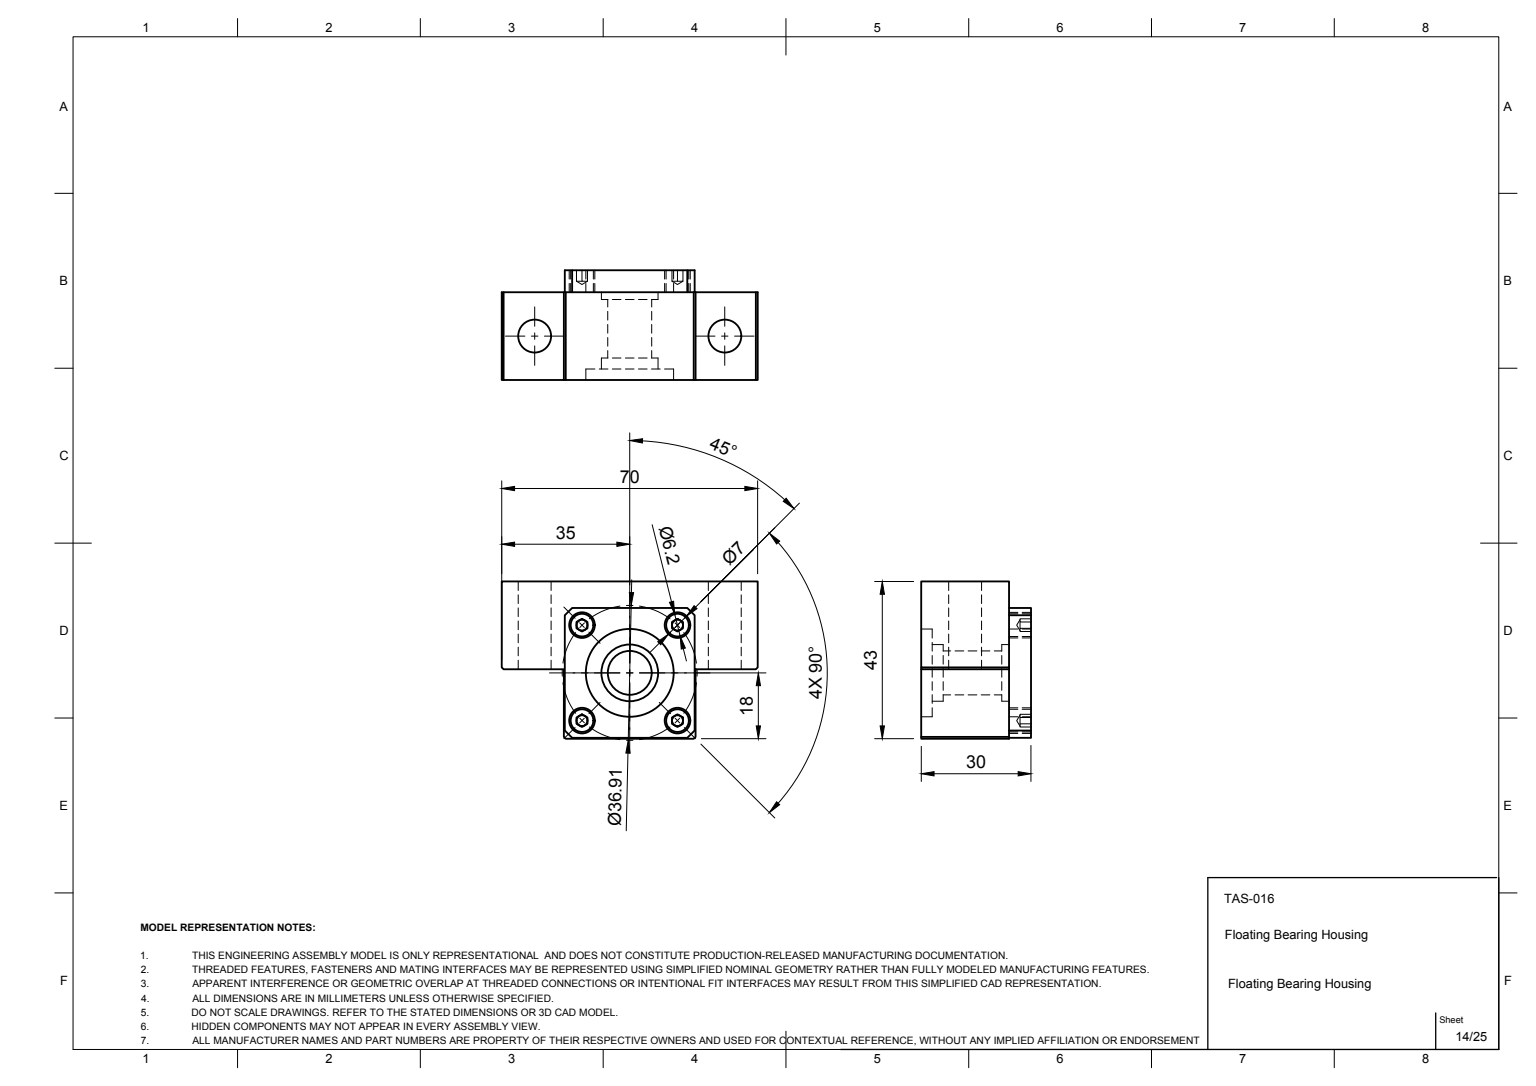
ISO-10303-21;
HEADER;
/* Generated by software containing ST-Developer
 * from STEP Tools, Inc. (www.steptools.com) 
 */

FILE_DESCRIPTION(
/* description */ ('STEP AP214'),
/* implementation_level */ '2;1');

FILE_NAME(
/* name */ 'Floating Bearing Housing.step',
/* time_stamp */ '2026-11-15T14:55:55-08:00',
/* author */ (''),
/* organization */ (''),
/* preprocessor_version */ 'ST-DEVELOPER v20.2',
/* originating_system */ 'Autodesk Translation Framework v15.17.0.0',
/* authorisation */ '');

FILE_SCHEMA (('AUTOMOTIVE_DESIGN { 1 0 10303 214 3 1 1 }'));
ENDSEC;

DATA;
#10=MECHANICAL_DESIGN_GEOMETRIC_PRESENTATION_REPRESENTATION('',(#929),#57079);
#871=SHAPE_REPRESENTATION_RELATIONSHIP('SRR','None',#57256,#900);
#900=ADVANCED_BREP_SHAPE_REPRESENTATION('',(#966),#57048);
#929=STYLED_ITEM('',(#57444),#966);
#966=MANIFOLD_SOLID_BREP('Body1',#24529);
#1046=FACE_BOUND('',#3680,.T.);
#1047=FACE_BOUND('',#3682,.T.);
#1048=FACE_BOUND('',#3684,.T.);
#1049=FACE_BOUND('',#3686,.T.);
#1050=FACE_BOUND('',#3688,.T.);
#1051=FACE_BOUND('',#3690,.T.);
#1052=FACE_BOUND('',#3694,.T.);
#1053=FACE_BOUND('',#3695,.T.);
#1054=FACE_BOUND('',#3699,.T.);
#1055=FACE_BOUND('',#3706,.T.);
#1056=FACE_BOUND('',#3708,.T.);
#1057=FACE_BOUND('',#3709,.T.);
#1058=FACE_BOUND('',#3710,.T.);
#1059=FACE_BOUND('',#3711,.T.);
#1060=FACE_BOUND('',#3712,.T.);
#1061=FACE_BOUND('',#3722,.T.);
#1062=FACE_BOUND('',#3724,.T.);
#1063=FACE_BOUND('',#3726,.T.);
#1064=FACE_BOUND('',#3728,.T.);
#1065=FACE_BOUND('',#3778,.T.);
#1066=FACE_BOUND('',#3780,.T.);
#1067=FACE_BOUND('',#3782,.T.);
#1068=FACE_BOUND('',#3784,.T.);
#1371=PLANE('',#25131);
#1372=PLANE('',#25132);
#1373=PLANE('',#25133);
#1374=PLANE('',#25134);
#1375=PLANE('',#25135);
#1376=PLANE('',#25136);
#1377=PLANE('',#25137);
#1378=PLANE('',#25138);
#1379=PLANE('',#25139);
#1380=PLANE('',#25140);
#1381=PLANE('',#25141);
#1382=PLANE('',#25142);
#1383=PLANE('',#25143);
#1384=PLANE('',#25144);
#1385=PLANE('',#25145);
#1386=PLANE('',#25146);
#1387=PLANE('',#25147);
#1388=PLANE('',#25148);
#1389=PLANE('',#25149);
#1390=PLANE('',#25150);
#1391=PLANE('',#25151);
#1392=PLANE('',#25152);
#1393=PLANE('',#25153);
#1394=PLANE('',#25154);
#1395=PLANE('',#25155);
#1396=PLANE('',#25156);
#1397=PLANE('',#25157);
#1398=PLANE('',#25158);
#1399=PLANE('',#25159);
#1400=PLANE('',#25160);
#1401=PLANE('',#25161);
#1402=PLANE('',#25162);
#1403=PLANE('',#25163);
#1404=PLANE('',#25164);
#1405=PLANE('',#25165);
#1406=PLANE('',#25166);
#1407=PLANE('',#25167);
#1408=PLANE('',#25168);
#1409=PLANE('',#25169);
#1410=PLANE('',#25170);
#1411=PLANE('',#25171);
#1412=PLANE('',#25172);
#1413=PLANE('',#25173);
#1414=PLANE('',#25174);
#1415=PLANE('',#25175);
#1416=PLANE('',#25176);
#1417=PLANE('',#25177);
#1418=PLANE('',#25178);
#1419=PLANE('',#25179);
#1420=PLANE('',#25180);
#1421=PLANE('',#25181);
#1422=PLANE('',#25182);
#1423=PLANE('',#25183);
#1424=PLANE('',#25184);
#1425=PLANE('',#25185);
#1426=PLANE('',#25186);
#1427=PLANE('',#25187);
#1428=PLANE('',#25188);
#1429=PLANE('',#25189);
#1430=PLANE('',#25190);
#1431=PLANE('',#25191);
#1432=PLANE('',#25192);
#1433=PLANE('',#25193);
#1434=PLANE('',#25194);
#1435=PLANE('',#25195);
#1436=PLANE('',#25196);
#1437=PLANE('',#25197);
#1438=PLANE('',#25198);
#1439=PLANE('',#25199);
#1440=PLANE('',#25200);
#1441=PLANE('',#25201);
#1442=PLANE('',#25202);
#1443=PLANE('',#25203);
#1444=PLANE('',#25204);
#1445=PLANE('',#25205);
#1446=PLANE('',#25206);
#1447=PLANE('',#25207);
#1448=PLANE('',#25208);
#1449=PLANE('',#25209);
#1450=PLANE('',#25210);
#1451=PLANE('',#25211);
#1452=PLANE('',#25212);
#1453=PLANE('',#25213);
#2114=CONICAL_SURFACE('',#25079,1.5,1.02974425867665);
#2115=CONICAL_SURFACE('',#25086,1.5,1.02974425867665);
#2116=CONICAL_SURFACE('',#25093,1.5,1.02974425867665);
#2117=CONICAL_SURFACE('',#25100,1.5,1.02974425867665);
#2239=FACE_OUTER_BOUND('',#3660,.T.);
#2240=FACE_OUTER_BOUND('',#3661,.T.);
#2241=FACE_OUTER_BOUND('',#3662,.T.);
#2242=FACE_OUTER_BOUND('',#3663,.T.);
#2243=FACE_OUTER_BOUND('',#3664,.T.);
#2244=FACE_OUTER_BOUND('',#3665,.T.);
#2245=FACE_OUTER_BOUND('',#3666,.T.);
#2246=FACE_OUTER_BOUND('',#3667,.T.);
#2247=FACE_OUTER_BOUND('',#3668,.T.);
#2248=FACE_OUTER_BOUND('',#3669,.T.);
#2249=FACE_OUTER_BOUND('',#3670,.T.);
#2250=FACE_OUTER_BOUND('',#3671,.T.);
#2251=FACE_OUTER_BOUND('',#3672,.T.);
#2252=FACE_OUTER_BOUND('',#3673,.T.);
#2253=FACE_OUTER_BOUND('',#3674,.T.);
#2254=FACE_OUTER_BOUND('',#3675,.T.);
#2255=FACE_OUTER_BOUND('',#3676,.T.);
#2256=FACE_OUTER_BOUND('',#3677,.T.);
#2257=FACE_OUTER_BOUND('',#3678,.T.);
#2258=FACE_OUTER_BOUND('',#3679,.T.);
#2259=FACE_OUTER_BOUND('',#3681,.T.);
#2260=FACE_OUTER_BOUND('',#3683,.T.);
#2261=FACE_OUTER_BOUND('',#3685,.T.);
#2262=FACE_OUTER_BOUND('',#3687,.T.);
#2263=FACE_OUTER_BOUND('',#3689,.T.);
#2264=FACE_OUTER_BOUND('',#3691,.T.);
#2265=FACE_OUTER_BOUND('',#3692,.T.);
#2266=FACE_OUTER_BOUND('',#3693,.T.);
#2267=FACE_OUTER_BOUND('',#3696,.T.);
#2268=FACE_OUTER_BOUND('',#3697,.T.);
#2269=FACE_OUTER_BOUND('',#3698,.T.);
#2270=FACE_OUTER_BOUND('',#3700,.T.);
#2271=FACE_OUTER_BOUND('',#3701,.T.);
#2272=FACE_OUTER_BOUND('',#3702,.T.);
#2273=FACE_OUTER_BOUND('',#3703,.T.);
#2274=FACE_OUTER_BOUND('',#3704,.T.);
#2275=FACE_OUTER_BOUND('',#3705,.T.);
#2276=FACE_OUTER_BOUND('',#3707,.T.);
#2277=FACE_OUTER_BOUND('',#3713,.T.);
#2278=FACE_OUTER_BOUND('',#3714,.T.);
#2279=FACE_OUTER_BOUND('',#3715,.T.);
#2280=FACE_OUTER_BOUND('',#3716,.T.);
#2281=FACE_OUTER_BOUND('',#3717,.T.);
#2282=FACE_OUTER_BOUND('',#3718,.T.);
#2283=FACE_OUTER_BOUND('',#3719,.T.);
#2284=FACE_OUTER_BOUND('',#3720,.T.);
#2285=FACE_OUTER_BOUND('',#3721,.T.);
#2286=FACE_OUTER_BOUND('',#3723,.T.);
#2287=FACE_OUTER_BOUND('',#3725,.T.);
#2288=FACE_OUTER_BOUND('',#3727,.T.);
#2289=FACE_OUTER_BOUND('',#3729,.T.);
#2290=FACE_OUTER_BOUND('',#3730,.T.);
#2291=FACE_OUTER_BOUND('',#3731,.T.);
#2292=FACE_OUTER_BOUND('',#3732,.T.);
#2293=FACE_OUTER_BOUND('',#3733,.T.);
#2294=FACE_OUTER_BOUND('',#3734,.T.);
#2295=FACE_OUTER_BOUND('',#3735,.T.);
#2296=FACE_OUTER_BOUND('',#3736,.T.);
#2297=FACE_OUTER_BOUND('',#3737,.T.);
#2298=FACE_OUTER_BOUND('',#3738,.T.);
#2299=FACE_OUTER_BOUND('',#3739,.T.);
#2300=FACE_OUTER_BOUND('',#3740,.T.);
#2301=FACE_OUTER_BOUND('',#3741,.T.);
#2302=FACE_OUTER_BOUND('',#3742,.T.);
#2303=FACE_OUTER_BOUND('',#3743,.T.);
#2304=FACE_OUTER_BOUND('',#3744,.T.);
#2305=FACE_OUTER_BOUND('',#3745,.T.);
#2306=FACE_OUTER_BOUND('',#3746,.T.);
#2307=FACE_OUTER_BOUND('',#3747,.T.);
#2308=FACE_OUTER_BOUND('',#3748,.T.);
#2309=FACE_OUTER_BOUND('',#3749,.T.);
#2310=FACE_OUTER_BOUND('',#3750,.T.);
#2311=FACE_OUTER_BOUND('',#3751,.T.);
#2312=FACE_OUTER_BOUND('',#3752,.T.);
#2313=FACE_OUTER_BOUND('',#3753,.T.);
#2314=FACE_OUTER_BOUND('',#3754,.T.);
#2315=FACE_OUTER_BOUND('',#3755,.T.);
#2316=FACE_OUTER_BOUND('',#3756,.T.);
#2317=FACE_OUTER_BOUND('',#3757,.T.);
#2318=FACE_OUTER_BOUND('',#3758,.T.);
#2319=FACE_OUTER_BOUND('',#3759,.T.);
#2320=FACE_OUTER_BOUND('',#3760,.T.);
#2321=FACE_OUTER_BOUND('',#3761,.T.);
#2322=FACE_OUTER_BOUND('',#3762,.T.);
#2323=FACE_OUTER_BOUND('',#3763,.T.);
#2324=FACE_OUTER_BOUND('',#3764,.T.);
#2325=FACE_OUTER_BOUND('',#3765,.T.);
#2326=FACE_OUTER_BOUND('',#3766,.T.);
#2327=FACE_OUTER_BOUND('',#3767,.T.);
#2328=FACE_OUTER_BOUND('',#3768,.T.);
#2329=FACE_OUTER_BOUND('',#3769,.T.);
#2330=FACE_OUTER_BOUND('',#3770,.T.);
#2331=FACE_OUTER_BOUND('',#3771,.T.);
#2332=FACE_OUTER_BOUND('',#3772,.T.);
#2333=FACE_OUTER_BOUND('',#3773,.T.);
#2334=FACE_OUTER_BOUND('',#3774,.T.);
#2335=FACE_OUTER_BOUND('',#3775,.T.);
#2336=FACE_OUTER_BOUND('',#3776,.T.);
#2337=FACE_OUTER_BOUND('',#3777,.T.);
#2338=FACE_OUTER_BOUND('',#3779,.T.);
#2339=FACE_OUTER_BOUND('',#3781,.T.);
#2340=FACE_OUTER_BOUND('',#3783,.T.);
#3660=EDGE_LOOP('',(#16272,#16273,#16274,#16275));
#3661=EDGE_LOOP('',(#16276,#16277,#16278,#16279));
#3662=EDGE_LOOP('',(#16280,#16281,#16282,#16283));
#3663=EDGE_LOOP('',(#16284,#16285,#16286,#16287));
#3664=EDGE_LOOP('',(#16288,#16289,#16290,#16291));
#3665=EDGE_LOOP('',(#16292,#16293,#16294,#16295));
#3666=EDGE_LOOP('',(#16296,#16297,#16298,#16299));
#3667=EDGE_LOOP('',(#16300,#16301,#16302,#16303,#16304,#16305,#16306,#16307));
#3668=EDGE_LOOP('',(#16308,#16309,#16310,#16311,#16312,#16313,#16314,#16315));
#3669=EDGE_LOOP('',(#16316,#16317,#16318,#16319,#16320,#16321,#16322,#16323));
#3670=EDGE_LOOP('',(#16324,#16325,#16326,#16327,#16328,#16329,#16330,#16331));
#3671=EDGE_LOOP('',(#16332,#16333,#16334,#16335));
#3672=EDGE_LOOP('',(#16336,#16337,#16338,#16339));
#3673=EDGE_LOOP('',(#16340,#16341,#16342,#16343));
#3674=EDGE_LOOP('',(#16344,#16345,#16346,#16347));
#3675=EDGE_LOOP('',(#16348,#16349,#16350,#16351));
#3676=EDGE_LOOP('',(#16352,#16353,#16354,#16355));
#3677=EDGE_LOOP('',(#16356,#16357,#16358,#16359));
#3678=EDGE_LOOP('',(#16360,#16361,#16362,#16363));
#3679=EDGE_LOOP('',(#16364));
#3680=EDGE_LOOP('',(#16365));
#3681=EDGE_LOOP('',(#16366));
#3682=EDGE_LOOP('',(#16367));
#3683=EDGE_LOOP('',(#16368));
#3684=EDGE_LOOP('',(#16369));
#3685=EDGE_LOOP('',(#16370));
#3686=EDGE_LOOP('',(#16371));
#3687=EDGE_LOOP('',(#16372,#16373,#16374,#16375,#16376,#16377,#16378,#16379,
#16380,#16381,#16382,#16383));
#3688=EDGE_LOOP('',(#16384,#16385,#16386,#16387,#16388,#16389,#16390,#16391));
#3689=EDGE_LOOP('',(#16392,#16393,#16394,#16395));
#3690=EDGE_LOOP('',(#16396));
#3691=EDGE_LOOP('',(#16397,#16398,#16399,#16400));
#3692=EDGE_LOOP('',(#16401,#16402,#16403,#16404));
#3693=EDGE_LOOP('',(#16405,#16406,#16407,#16408));
#3694=EDGE_LOOP('',(#16409));
#3695=EDGE_LOOP('',(#16410));
#3696=EDGE_LOOP('',(#16411,#16412,#16413,#16414));
#3697=EDGE_LOOP('',(#16415,#16416,#16417,#16418));
#3698=EDGE_LOOP('',(#16419,#16420,#16421,#16422));
#3699=EDGE_LOOP('',(#16423));
#3700=EDGE_LOOP('',(#16424,#16425,#16426,#16427));
#3701=EDGE_LOOP('',(#16428,#16429,#16430,#16431));
#3702=EDGE_LOOP('',(#16432,#16433,#16434,#16435));
#3703=EDGE_LOOP('',(#16436,#16437,#16438,#16439));
#3704=EDGE_LOOP('',(#16440,#16441,#16442,#16443));
#3705=EDGE_LOOP('',(#16444,#16445,#16446,#16447,#16448,#16449,#16450,#16451,
#16452,#16453,#16454,#16455));
#3706=EDGE_LOOP('',(#16456));
#3707=EDGE_LOOP('',(#16457,#16458,#16459,#16460,#16461,#16462,#16463,#16464));
#3708=EDGE_LOOP('',(#16465));
#3709=EDGE_LOOP('',(#16466));
#3710=EDGE_LOOP('',(#16467));
#3711=EDGE_LOOP('',(#16468));
#3712=EDGE_LOOP('',(#16469));
#3713=EDGE_LOOP('',(#16470,#16471,#16472,#16473));
#3714=EDGE_LOOP('',(#16474,#16475,#16476,#16477));
#3715=EDGE_LOOP('',(#16478,#16479,#16480,#16481));
#3716=EDGE_LOOP('',(#16482,#16483,#16484,#16485));
#3717=EDGE_LOOP('',(#16486,#16487,#16488,#16489));
#3718=EDGE_LOOP('',(#16490,#16491,#16492,#16493));
#3719=EDGE_LOOP('',(#16494,#16495,#16496,#16497));
#3720=EDGE_LOOP('',(#16498,#16499,#16500,#16501));
#3721=EDGE_LOOP('',(#16502));
#3722=EDGE_LOOP('',(#16503,#16504,#16505,#16506,#16507,#16508));
#3723=EDGE_LOOP('',(#16509));
#3724=EDGE_LOOP('',(#16510,#16511,#16512,#16513,#16514,#16515));
#3725=EDGE_LOOP('',(#16516));
#3726=EDGE_LOOP('',(#16517,#16518,#16519,#16520,#16521,#16522));
#3727=EDGE_LOOP('',(#16523));
#3728=EDGE_LOOP('',(#16524,#16525,#16526,#16527,#16528,#16529));
#3729=EDGE_LOOP('',(#16530,#16531,#16532,#16533,#16534));
#3730=EDGE_LOOP('',(#16535,#16536,#16537,#16538,#16539));
#3731=EDGE_LOOP('',(#16540,#16541,#16542,#16543,#16544));
#3732=EDGE_LOOP('',(#16545,#16546,#16547,#16548,#16549));
#3733=EDGE_LOOP('',(#16550,#16551,#16552,#16553,#16554));
#3734=EDGE_LOOP('',(#16555,#16556,#16557,#16558,#16559));
#3735=EDGE_LOOP('',(#16560,#16561,#16562));
#3736=EDGE_LOOP('',(#16563,#16564,#16565));
#3737=EDGE_LOOP('',(#16566,#16567,#16568));
#3738=EDGE_LOOP('',(#16569,#16570,#16571));
#3739=EDGE_LOOP('',(#16572,#16573,#16574));
#3740=EDGE_LOOP('',(#16575,#16576,#16577));
#3741=EDGE_LOOP('',(#16578,#16579,#16580,#16581,#16582));
#3742=EDGE_LOOP('',(#16583,#16584,#16585,#16586,#16587));
#3743=EDGE_LOOP('',(#16588,#16589,#16590,#16591,#16592));
#3744=EDGE_LOOP('',(#16593,#16594,#16595,#16596,#16597));
#3745=EDGE_LOOP('',(#16598,#16599,#16600,#16601,#16602));
#3746=EDGE_LOOP('',(#16603,#16604,#16605,#16606,#16607));
#3747=EDGE_LOOP('',(#16608,#16609,#16610));
#3748=EDGE_LOOP('',(#16611,#16612,#16613));
#3749=EDGE_LOOP('',(#16614,#16615,#16616));
#3750=EDGE_LOOP('',(#16617,#16618,#16619));
#3751=EDGE_LOOP('',(#16620,#16621,#16622));
#3752=EDGE_LOOP('',(#16623,#16624,#16625));
#3753=EDGE_LOOP('',(#16626,#16627,#16628,#16629,#16630));
#3754=EDGE_LOOP('',(#16631,#16632,#16633,#16634,#16635));
#3755=EDGE_LOOP('',(#16636,#16637,#16638,#16639,#16640));
#3756=EDGE_LOOP('',(#16641,#16642,#16643,#16644,#16645));
#3757=EDGE_LOOP('',(#16646,#16647,#16648,#16649,#16650));
#3758=EDGE_LOOP('',(#16651,#16652,#16653,#16654,#16655));
#3759=EDGE_LOOP('',(#16656,#16657,#16658));
#3760=EDGE_LOOP('',(#16659,#16660,#16661));
#3761=EDGE_LOOP('',(#16662,#16663,#16664));
#3762=EDGE_LOOP('',(#16665,#16666,#16667));
#3763=EDGE_LOOP('',(#16668,#16669,#16670));
#3764=EDGE_LOOP('',(#16671,#16672,#16673));
#3765=EDGE_LOOP('',(#16674,#16675,#16676,#16677,#16678));
#3766=EDGE_LOOP('',(#16679,#16680,#16681,#16682,#16683));
#3767=EDGE_LOOP('',(#16684,#16685,#16686,#16687,#16688));
#3768=EDGE_LOOP('',(#16689,#16690,#16691,#16692,#16693));
#3769=EDGE_LOOP('',(#16694,#16695,#16696,#16697,#16698));
#3770=EDGE_LOOP('',(#16699,#16700,#16701,#16702,#16703));
#3771=EDGE_LOOP('',(#16704,#16705,#16706));
#3772=EDGE_LOOP('',(#16707,#16708,#16709));
#3773=EDGE_LOOP('',(#16710,#16711,#16712));
#3774=EDGE_LOOP('',(#16713,#16714,#16715));
#3775=EDGE_LOOP('',(#16716,#16717,#16718));
#3776=EDGE_LOOP('',(#16719,#16720,#16721));
#3777=EDGE_LOOP('',(#16722));
#3778=EDGE_LOOP('',(#16723));
#3779=EDGE_LOOP('',(#16724));
#3780=EDGE_LOOP('',(#16725));
#3781=EDGE_LOOP('',(#16726));
#3782=EDGE_LOOP('',(#16727));
#3783=EDGE_LOOP('',(#16728));
#3784=EDGE_LOOP('',(#16729));
#5331=LINE('',#35183,#7298);
#5332=LINE('',#35189,#7299);
#5333=LINE('',#35195,#7300);
#5334=LINE('',#35201,#7301);
#5335=LINE('',#35207,#7302);
#5336=LINE('',#35213,#7303);
#5337=LINE('',#35219,#7304);
#5338=LINE('',#35224,#7305);
#5339=LINE('',#35239,#7306);
#5340=LINE('',#35254,#7307);
#5341=LINE('',#35269,#7308);
#5342=LINE('',#35285,#7309);
#5343=LINE('',#35291,#7310);
#5344=LINE('',#35297,#7311);
#5345=LINE('',#35303,#7312);
#5346=LINE('',#35309,#7313);
#5347=LINE('',#35315,#7314);
#5348=LINE('',#35321,#7315);
#5349=LINE('',#35327,#7316);
#5350=LINE('',#35336,#7317);
#5351=LINE('',#35338,#7318);
#5352=LINE('',#35340,#7319);
#5353=LINE('',#35342,#7320);
#5354=LINE('',#35344,#7321);
#5355=LINE('',#35346,#7322);
#5356=LINE('',#35348,#7323);
#5357=LINE('',#35350,#7324);
#5358=LINE('',#35352,#7325);
#5359=LINE('',#35354,#7326);
#5360=LINE('',#35356,#7327);
#5361=LINE('',#35357,#7328);
#5362=LINE('',#35360,#7329);
#5363=LINE('',#35362,#7330);
#5364=LINE('',#35364,#7331);
#5365=LINE('',#35366,#7332);
#5366=LINE('',#35368,#7333);
#5367=LINE('',#35370,#7334);
#5368=LINE('',#35372,#7335);
#5369=LINE('',#35373,#7336);
#5370=LINE('',#35377,#7337);
#5371=LINE('',#35378,#7338);
#5372=LINE('',#35379,#7339);
#5373=LINE('',#35382,#7340);
#5374=LINE('',#35383,#7341);
#5375=LINE('',#35386,#7342);
#5376=LINE('',#35387,#7343);
#5377=LINE('',#35390,#7344);
#5378=LINE('',#35391,#7345);
#5379=LINE('',#35394,#7346);
#5380=LINE('',#35395,#7347);
#5381=LINE('',#35398,#7348);
#5382=LINE('',#35399,#7349);
#5383=LINE('',#35402,#7350);
#5384=LINE('',#35403,#7351);
#5385=LINE('',#35406,#7352);
#5386=LINE('',#35407,#7353);
#5387=LINE('',#35410,#7354);
#5388=LINE('',#35411,#7355);
#5389=LINE('',#35414,#7356);
#5390=LINE('',#35415,#7357);
#5391=LINE('',#35418,#7358);
#5392=LINE('',#35419,#7359);
#5393=LINE('',#35421,#7360);
#5394=LINE('',#35426,#7361);
#5395=LINE('',#35428,#7362);
#5396=LINE('',#35430,#7363);
#5397=LINE('',#35432,#7364);
#5398=LINE('',#35434,#7365);
#5399=LINE('',#35436,#7366);
#5400=LINE('',#35438,#7367);
#5401=LINE('',#35439,#7368);
#5402=LINE('',#35441,#7369);
#5403=LINE('',#35442,#7370);
#5404=LINE('',#35444,#7371);
#5405=LINE('',#35446,#7372);
#5406=LINE('',#35448,#7373);
#5407=LINE('',#35450,#7374);
#5408=LINE('',#35452,#7375);
#5409=LINE('',#35454,#7376);
#5410=LINE('',#35459,#7377);
#5411=LINE('',#35461,#7378);
#5412=LINE('',#35463,#7379);
#5413=LINE('',#35465,#7380);
#5414=LINE('',#35467,#7381);
#5415=LINE('',#35468,#7382);
#5416=LINE('',#35472,#7383);
#5417=LINE('',#35474,#7384);
#5418=LINE('',#35476,#7385);
#5419=LINE('',#35478,#7386);
#5420=LINE('',#35480,#7387);
#5421=LINE('',#35481,#7388);
#5422=LINE('',#35485,#7389);
#5423=LINE('',#35487,#7390);
#5424=LINE('',#35489,#7391);
#5425=LINE('',#35491,#7392);
#5426=LINE('',#35493,#7393);
#5427=LINE('',#35494,#7394);
#5428=LINE('',#35498,#7395);
#5429=LINE('',#35500,#7396);
#5430=LINE('',#35502,#7397);
#5431=LINE('',#35504,#7398);
#5432=LINE('',#35506,#7399);
#5433=LINE('',#35507,#7400);
#5434=LINE('',#35510,#7401);
#5435=LINE('',#35511,#7402);
#5436=LINE('',#35513,#7403);
#5437=LINE('',#35514,#7404);
#5438=LINE('',#35516,#7405);
#5439=LINE('',#35518,#7406);
#5440=LINE('',#35519,#7407);
#5441=LINE('',#35521,#7408);
#5442=LINE('',#35523,#7409);
#5443=LINE('',#35524,#7410);
#5444=LINE('',#35526,#7411);
#5445=LINE('',#35528,#7412);
#5446=LINE('',#35529,#7413);
#5447=LINE('',#35531,#7414);
#5448=LINE('',#35533,#7415);
#5449=LINE('',#35534,#7416);
#5450=LINE('',#35536,#7417);
#5451=LINE('',#35537,#7418);
#5452=LINE('',#35546,#7419);
#5453=LINE('',#35547,#7420);
#5454=LINE('',#35549,#7421);
#5455=LINE('',#35550,#7422);
#5456=LINE('',#35552,#7423);
#5457=LINE('',#35554,#7424);
#5458=LINE('',#35555,#7425);
#5459=LINE('',#35557,#7426);
#5460=LINE('',#35559,#7427);
#5461=LINE('',#35560,#7428);
#5462=LINE('',#35562,#7429);
#5463=LINE('',#35564,#7430);
#5464=LINE('',#35565,#7431);
#5465=LINE('',#35567,#7432);
#5466=LINE('',#35569,#7433);
#5467=LINE('',#35570,#7434);
#5468=LINE('',#35572,#7435);
#5469=LINE('',#35573,#7436);
#5470=LINE('',#35582,#7437);
#5471=LINE('',#35583,#7438);
#5472=LINE('',#35585,#7439);
#5473=LINE('',#35586,#7440);
#5474=LINE('',#35588,#7441);
#5475=LINE('',#35590,#7442);
#5476=LINE('',#35591,#7443);
#5477=LINE('',#35593,#7444);
#5478=LINE('',#35595,#7445);
#5479=LINE('',#35596,#7446);
#5480=LINE('',#35598,#7447);
#5481=LINE('',#35600,#7448);
#5482=LINE('',#35601,#7449);
#5483=LINE('',#35603,#7450);
#5484=LINE('',#35605,#7451);
#5485=LINE('',#35606,#7452);
#5486=LINE('',#35608,#7453);
#5487=LINE('',#35609,#7454);
#5488=LINE('',#35618,#7455);
#5489=LINE('',#35619,#7456);
#5490=LINE('',#35621,#7457);
#5491=LINE('',#35622,#7458);
#5492=LINE('',#35624,#7459);
#5493=LINE('',#35626,#7460);
#5494=LINE('',#35627,#7461);
#5495=LINE('',#35629,#7462);
#5496=LINE('',#35631,#7463);
#5497=LINE('',#35632,#7464);
#5498=LINE('',#35634,#7465);
#5499=LINE('',#35636,#7466);
#5500=LINE('',#35637,#7467);
#5501=LINE('',#35639,#7468);
#5502=LINE('',#35641,#7469);
#5503=LINE('',#35642,#7470);
#5504=LINE('',#35644,#7471);
#5505=LINE('',#35645,#7472);
#7298=VECTOR('',#27911,4.49999999999999);
#7299=VECTOR('',#27918,4.49999999999999);
#7300=VECTOR('',#27925,12.);
#7301=VECTOR('',#27932,7.75);
#7302=VECTOR('',#27939,6.);
#7303=VECTOR('',#27946,7.74999999999999);
#7304=VECTOR('',#27953,12.);
#7305=VECTOR('',#27958,1.5);
#7306=VECTOR('',#27973,1.5);
#7307=VECTOR('',#27988,1.5);
#7308=VECTOR('',#28003,1.5);
#7309=VECTOR('',#28020,3.1);
#7310=VECTOR('',#28027,3.1);
#7311=VECTOR('',#28034,3.1);
#7312=VECTOR('',#28041,3.1);
#7313=VECTOR('',#28048,3.5);
#7314=VECTOR('',#28055,3.5);
#7315=VECTOR('',#28062,3.50000000000001);
#7316=VECTOR('',#28069,3.50000000000001);
#7317=VECTOR('',#28082,1000.);
#7318=VECTOR('',#28083,1000.);
#7319=VECTOR('',#28084,1000.);
#7320=VECTOR('',#28085,1000.);
#7321=VECTOR('',#28086,1000.);
#7322=VECTOR('',#28087,1000.);
#7323=VECTOR('',#28088,1000.);
#7324=VECTOR('',#28089,1000.);
#7325=VECTOR('',#28090,1000.);
#7326=VECTOR('',#28091,1000.);
#7327=VECTOR('',#28092,1000.);
#7328=VECTOR('',#28093,1000.);
#7329=VECTOR('',#28094,1000.);
#7330=VECTOR('',#28095,1000.);
#7331=VECTOR('',#28096,1000.);
#7332=VECTOR('',#28097,1000.);
#7333=VECTOR('',#28098,1000.);
#7334=VECTOR('',#28099,1000.);
#7335=VECTOR('',#28100,1000.);
#7336=VECTOR('',#28101,1000.);
#7337=VECTOR('',#28104,1000.);
#7338=VECTOR('',#28105,1000.);
#7339=VECTOR('',#28106,1000.);
#7340=VECTOR('',#28109,1000.);
#7341=VECTOR('',#28110,1000.);
#7342=VECTOR('',#28113,1000.);
#7343=VECTOR('',#28114,1000.);
#7344=VECTOR('',#28117,1000.);
#7345=VECTOR('',#28118,1000.);
#7346=VECTOR('',#28121,1000.);
#7347=VECTOR('',#28122,1000.);
#7348=VECTOR('',#28125,1000.);
#7349=VECTOR('',#28126,1000.);
#7350=VECTOR('',#28129,1000.);
#7351=VECTOR('',#28130,1000.);
#7352=VECTOR('',#28133,1000.);
#7353=VECTOR('',#28134,1000.);
#7354=VECTOR('',#28137,1000.);
#7355=VECTOR('',#28138,1000.);
#7356=VECTOR('',#28141,1000.);
#7357=VECTOR('',#28142,1000.);
#7358=VECTOR('',#28145,1000.);
#7359=VECTOR('',#28146,1000.);
#7360=VECTOR('',#28149,1000.);
#7361=VECTOR('',#28154,1000.);
#7362=VECTOR('',#28155,1000.);
#7363=VECTOR('',#28156,1000.);
#7364=VECTOR('',#28157,1000.);
#7365=VECTOR('',#28158,1000.);
#7366=VECTOR('',#28159,1000.);
#7367=VECTOR('',#28160,1000.);
#7368=VECTOR('',#28161,1000.);
#7369=VECTOR('',#28164,1000.);
#7370=VECTOR('',#28165,1000.);
#7371=VECTOR('',#28168,1000.);
#7372=VECTOR('',#28171,1000.);
#7373=VECTOR('',#28174,1000.);
#7374=VECTOR('',#28177,1000.);
#7375=VECTOR('',#28180,1000.);
#7376=VECTOR('',#28183,1000.);
#7377=VECTOR('',#28188,1000.);
#7378=VECTOR('',#28189,1000.);
#7379=VECTOR('',#28190,1000.);
#7380=VECTOR('',#28191,1000.);
#7381=VECTOR('',#28192,1000.);
#7382=VECTOR('',#28193,1000.);
#7383=VECTOR('',#28196,1000.);
#7384=VECTOR('',#28197,1000.);
#7385=VECTOR('',#28198,1000.);
#7386=VECTOR('',#28199,1000.);
#7387=VECTOR('',#28200,1000.);
#7388=VECTOR('',#28201,1000.);
#7389=VECTOR('',#28204,1000.);
#7390=VECTOR('',#28205,1000.);
#7391=VECTOR('',#28206,1000.);
#7392=VECTOR('',#28207,1000.);
#7393=VECTOR('',#28208,1000.);
#7394=VECTOR('',#28209,1000.);
#7395=VECTOR('',#28212,1000.);
#7396=VECTOR('',#28213,1000.);
#7397=VECTOR('',#28214,1000.);
#7398=VECTOR('',#28215,1000.);
#7399=VECTOR('',#28216,1000.);
#7400=VECTOR('',#28217,1000.);
#7401=VECTOR('',#28220,1000.);
#7402=VECTOR('',#28221,1000.);
#7403=VECTOR('',#28222,1000.);
#7404=VECTOR('',#28223,1000.);
#7405=VECTOR('',#28226,1000.);
#7406=VECTOR('',#28227,1000.);
#7407=VECTOR('',#28228,1000.);
#7408=VECTOR('',#28231,1000.);
#7409=VECTOR('',#28232,1000.);
#7410=VECTOR('',#28233,1000.);
#7411=VECTOR('',#28236,1000.);
#7412=VECTOR('',#28237,1000.);
#7413=VECTOR('',#28238,1000.);
#7414=VECTOR('',#28241,1000.);
#7415=VECTOR('',#28242,1000.);
#7416=VECTOR('',#28243,1000.);
#7417=VECTOR('',#28246,1000.);
#7418=VECTOR('',#28247,1000.);
#7419=VECTOR('',#28262,1000.);
#7420=VECTOR('',#28263,1000.);
#7421=VECTOR('',#28264,1000.);
#7422=VECTOR('',#28265,1000.);
#7423=VECTOR('',#28268,1000.);
#7424=VECTOR('',#28269,1000.);
#7425=VECTOR('',#28270,1000.);
#7426=VECTOR('',#28273,1000.);
#7427=VECTOR('',#28274,1000.);
#7428=VECTOR('',#28275,1000.);
#7429=VECTOR('',#28278,1000.);
#7430=VECTOR('',#28279,1000.);
#7431=VECTOR('',#28280,1000.);
#7432=VECTOR('',#28283,1000.);
#7433=VECTOR('',#28284,1000.);
#7434=VECTOR('',#28285,1000.);
#7435=VECTOR('',#28288,1000.);
#7436=VECTOR('',#28289,1000.);
#7437=VECTOR('',#28304,1000.);
#7438=VECTOR('',#28305,1000.);
#7439=VECTOR('',#28306,1000.);
#7440=VECTOR('',#28307,1000.);
#7441=VECTOR('',#28310,1000.);
#7442=VECTOR('',#28311,1000.);
#7443=VECTOR('',#28312,1000.);
#7444=VECTOR('',#28315,1000.);
#7445=VECTOR('',#28316,1000.);
#7446=VECTOR('',#28317,1000.);
#7447=VECTOR('',#28320,1000.);
#7448=VECTOR('',#28321,1000.);
#7449=VECTOR('',#28322,1000.);
#7450=VECTOR('',#28325,1000.);
#7451=VECTOR('',#28326,1000.);
#7452=VECTOR('',#28327,1000.);
#7453=VECTOR('',#28330,1000.);
#7454=VECTOR('',#28331,1000.);
#7455=VECTOR('',#28346,1000.);
#7456=VECTOR('',#28347,1000.);
#7457=VECTOR('',#28348,1000.);
#7458=VECTOR('',#28349,1000.);
#7459=VECTOR('',#28352,1000.);
#7460=VECTOR('',#28353,1000.);
#7461=VECTOR('',#28354,1000.);
#7462=VECTOR('',#28357,1000.);
#7463=VECTOR('',#28358,1000.);
#7464=VECTOR('',#28359,1000.);
#7465=VECTOR('',#28362,1000.);
#7466=VECTOR('',#28363,1000.);
#7467=VECTOR('',#28364,1000.);
#7468=VECTOR('',#28367,1000.);
#7469=VECTOR('',#28368,1000.);
#7470=VECTOR('',#28369,1000.);
#7471=VECTOR('',#28372,1000.);
#7472=VECTOR('',#28373,1000.);
#9270=CIRCLE('',#25059,4.5);
#9271=CIRCLE('',#25060,4.49999999999999);
#9272=CIRCLE('',#25062,4.5);
#9273=CIRCLE('',#25063,4.49999999999999);
#9274=CIRCLE('',#25065,12.);
#9275=CIRCLE('',#25066,12.);
#9276=CIRCLE('',#25068,7.75);
#9277=CIRCLE('',#25069,7.74999999999999);
#9278=CIRCLE('',#25071,6.00000000000001);
#9279=CIRCLE('',#25072,6.00000000000001);
#9280=CIRCLE('',#25074,7.74999999999999);
#9281=CIRCLE('',#25075,7.74999999999999);
#9282=CIRCLE('',#25077,12.);
#9283=CIRCLE('',#25078,12.);
#9284=CIRCLE('',#25080,1.5);
#9285=CIRCLE('',#25081,1.5);
#9286=CIRCLE('',#25082,1.5);
#9287=CIRCLE('',#25083,1.5);
#9288=CIRCLE('',#25084,1.5);
#9289=CIRCLE('',#25085,1.5);
#9290=CIRCLE('',#25087,1.5);
#9291=CIRCLE('',#25088,1.5);
#9292=CIRCLE('',#25089,1.5);
#9293=CIRCLE('',#25090,1.5);
#9294=CIRCLE('',#25091,1.5);
#9295=CIRCLE('',#25092,1.5);
#9296=CIRCLE('',#25094,1.5);
#9297=CIRCLE('',#25095,1.5);
#9298=CIRCLE('',#25096,1.5);
#9299=CIRCLE('',#25097,1.5);
#9300=CIRCLE('',#25098,1.5);
#9301=CIRCLE('',#25099,1.5);
#9302=CIRCLE('',#25101,1.5);
#9303=CIRCLE('',#25102,1.5);
#9304=CIRCLE('',#25103,1.5);
#9305=CIRCLE('',#25104,1.5);
#9306=CIRCLE('',#25105,1.5);
#9307=CIRCLE('',#25106,1.5);
#9308=CIRCLE('',#25108,3.1);
#9309=CIRCLE('',#25109,3.1);
#9310=CIRCLE('',#25111,3.1);
#9311=CIRCLE('',#25112,3.1);
#9312=CIRCLE('',#25114,3.1);
#9313=CIRCLE('',#25115,3.1);
#9314=CIRCLE('',#25117,3.1);
#9315=CIRCLE('',#25118,3.1);
#9316=CIRCLE('',#25120,3.5);
#9317=CIRCLE('',#25121,3.5);
#9318=CIRCLE('',#25123,3.5);
#9319=CIRCLE('',#25124,3.5);
#9320=CIRCLE('',#25126,3.50000000000001);
#9321=CIRCLE('',#25127,3.50000000000001);
#9322=CIRCLE('',#25129,3.50000000000001);
#9323=CIRCLE('',#25130,3.50000000000001);
#10397=VERTEX_POINT('',#35180);
#10398=VERTEX_POINT('',#35182);
#10399=VERTEX_POINT('',#35186);
#10400=VERTEX_POINT('',#35188);
#10401=VERTEX_POINT('',#35192);
#10402=VERTEX_POINT('',#35194);
#10403=VERTEX_POINT('',#35198);
#10404=VERTEX_POINT('',#35200);
#10405=VERTEX_POINT('',#35204);
#10406=VERTEX_POINT('',#35206);
#10407=VERTEX_POINT('',#35210);
#10408=VERTEX_POINT('',#35212);
#10409=VERTEX_POINT('',#35216);
#10410=VERTEX_POINT('',#35218);
#10411=VERTEX_POINT('',#35222);
#10412=VERTEX_POINT('',#35223);
#10413=VERTEX_POINT('',#35225);
#10414=VERTEX_POINT('',#35227);
#10415=VERTEX_POINT('',#35229);
#10416=VERTEX_POINT('',#35231);
#10417=VERTEX_POINT('',#35233);
#10418=VERTEX_POINT('',#35237);
#10419=VERTEX_POINT('',#35238);
#10420=VERTEX_POINT('',#35240);
#10421=VERTEX_POINT('',#35242);
#10422=VERTEX_POINT('',#35244);
#10423=VERTEX_POINT('',#35246);
#10424=VERTEX_POINT('',#35248);
#10425=VERTEX_POINT('',#35252);
#10426=VERTEX_POINT('',#35253);
#10427=VERTEX_POINT('',#35255);
#10428=VERTEX_POINT('',#35257);
#10429=VERTEX_POINT('',#35259);
#10430=VERTEX_POINT('',#35261);
#10431=VERTEX_POINT('',#35263);
#10432=VERTEX_POINT('',#35267);
#10433=VERTEX_POINT('',#35268);
#10434=VERTEX_POINT('',#35270);
#10435=VERTEX_POINT('',#35272);
#10436=VERTEX_POINT('',#35274);
#10437=VERTEX_POINT('',#35276);
#10438=VERTEX_POINT('',#35278);
#10439=VERTEX_POINT('',#35282);
#10440=VERTEX_POINT('',#35284);
#10441=VERTEX_POINT('',#35288);
#10442=VERTEX_POINT('',#35290);
#10443=VERTEX_POINT('',#35294);
#10444=VERTEX_POINT('',#35296);
#10445=VERTEX_POINT('',#35300);
#10446=VERTEX_POINT('',#35302);
#10447=VERTEX_POINT('',#35306);
#10448=VERTEX_POINT('',#35308);
#10449=VERTEX_POINT('',#35312);
#10450=VERTEX_POINT('',#35314);
#10451=VERTEX_POINT('',#35318);
#10452=VERTEX_POINT('',#35320);
#10453=VERTEX_POINT('',#35324);
#10454=VERTEX_POINT('',#35326);
#10455=VERTEX_POINT('',#35334);
#10456=VERTEX_POINT('',#35335);
#10457=VERTEX_POINT('',#35337);
#10458=VERTEX_POINT('',#35339);
#10459=VERTEX_POINT('',#35341);
#10460=VERTEX_POINT('',#35343);
#10461=VERTEX_POINT('',#35345);
#10462=VERTEX_POINT('',#35347);
#10463=VERTEX_POINT('',#35349);
#10464=VERTEX_POINT('',#35351);
#10465=VERTEX_POINT('',#35353);
#10466=VERTEX_POINT('',#35355);
#10467=VERTEX_POINT('',#35358);
#10468=VERTEX_POINT('',#35359);
#10469=VERTEX_POINT('',#35361);
#10470=VERTEX_POINT('',#35363);
#10471=VERTEX_POINT('',#35365);
#10472=VERTEX_POINT('',#35367);
#10473=VERTEX_POINT('',#35369);
#10474=VERTEX_POINT('',#35371);
#10475=VERTEX_POINT('',#35375);
#10476=VERTEX_POINT('',#35376);
#10477=VERTEX_POINT('',#35381);
#10478=VERTEX_POINT('',#35385);
#10479=VERTEX_POINT('',#35389);
#10480=VERTEX_POINT('',#35393);
#10481=VERTEX_POINT('',#35397);
#10482=VERTEX_POINT('',#35401);
#10483=VERTEX_POINT('',#35405);
#10484=VERTEX_POINT('',#35409);
#10485=VERTEX_POINT('',#35413);
#10486=VERTEX_POINT('',#35417);
#10487=VERTEX_POINT('',#35424);
#10488=VERTEX_POINT('',#35425);
#10489=VERTEX_POINT('',#35427);
#10490=VERTEX_POINT('',#35429);
#10491=VERTEX_POINT('',#35431);
#10492=VERTEX_POINT('',#35433);
#10493=VERTEX_POINT('',#35435);
#10494=VERTEX_POINT('',#35437);
#10495=VERTEX_POINT('',#35457);
#10496=VERTEX_POINT('',#35458);
#10497=VERTEX_POINT('',#35460);
#10498=VERTEX_POINT('',#35462);
#10499=VERTEX_POINT('',#35464);
#10500=VERTEX_POINT('',#35466);
#10501=VERTEX_POINT('',#35470);
#10502=VERTEX_POINT('',#35471);
#10503=VERTEX_POINT('',#35473);
#10504=VERTEX_POINT('',#35475);
#10505=VERTEX_POINT('',#35477);
#10506=VERTEX_POINT('',#35479);
#10507=VERTEX_POINT('',#35483);
#10508=VERTEX_POINT('',#35484);
#10509=VERTEX_POINT('',#35486);
#10510=VERTEX_POINT('',#35488);
#10511=VERTEX_POINT('',#35490);
#10512=VERTEX_POINT('',#35492);
#10513=VERTEX_POINT('',#35496);
#10514=VERTEX_POINT('',#35497);
#10515=VERTEX_POINT('',#35499);
#10516=VERTEX_POINT('',#35501);
#10517=VERTEX_POINT('',#35503);
#10518=VERTEX_POINT('',#35505);
#10519=VERTEX_POINT('',#35509);
#10520=VERTEX_POINT('',#35512);
#10521=VERTEX_POINT('',#35517);
#10522=VERTEX_POINT('',#35522);
#10523=VERTEX_POINT('',#35527);
#10524=VERTEX_POINT('',#35532);
#10525=VERTEX_POINT('',#35545);
#10526=VERTEX_POINT('',#35548);
#10527=VERTEX_POINT('',#35553);
#10528=VERTEX_POINT('',#35558);
#10529=VERTEX_POINT('',#35563);
#10530=VERTEX_POINT('',#35568);
#10531=VERTEX_POINT('',#35581);
#10532=VERTEX_POINT('',#35584);
#10533=VERTEX_POINT('',#35589);
#10534=VERTEX_POINT('',#35594);
#10535=VERTEX_POINT('',#35599);
#10536=VERTEX_POINT('',#35604);
#10537=VERTEX_POINT('',#35617);
#10538=VERTEX_POINT('',#35620);
#10539=VERTEX_POINT('',#35625);
#10540=VERTEX_POINT('',#35630);
#10541=VERTEX_POINT('',#35635);
#10542=VERTEX_POINT('',#35640);
#12681=EDGE_CURVE('',#10397,#10397,#9270,.T.);
#12682=EDGE_CURVE('',#10397,#10398,#5331,.T.);
#12683=EDGE_CURVE('',#10398,#10398,#9271,.T.);
#12684=EDGE_CURVE('',#10399,#10399,#9272,.T.);
#12685=EDGE_CURVE('',#10399,#10400,#5332,.T.);
#12686=EDGE_CURVE('',#10400,#10400,#9273,.T.);
#12687=EDGE_CURVE('',#10401,#10401,#9274,.T.);
#12688=EDGE_CURVE('',#10401,#10402,#5333,.T.);
#12689=EDGE_CURVE('',#10402,#10402,#9275,.T.);
#12690=EDGE_CURVE('',#10403,#10403,#9276,.T.);
#12691=EDGE_CURVE('',#10403,#10404,#5334,.T.);
#12692=EDGE_CURVE('',#10404,#10404,#9277,.T.);
#12693=EDGE_CURVE('',#10405,#10405,#9278,.T.);
#12694=EDGE_CURVE('',#10405,#10406,#5335,.T.);
#12695=EDGE_CURVE('',#10406,#10406,#9279,.T.);
#12696=EDGE_CURVE('',#10407,#10407,#9280,.T.);
#12697=EDGE_CURVE('',#10407,#10408,#5336,.T.);
#12698=EDGE_CURVE('',#10408,#10408,#9281,.T.);
#12699=EDGE_CURVE('',#10409,#10409,#9282,.T.);
#12700=EDGE_CURVE('',#10409,#10410,#5337,.T.);
#12701=EDGE_CURVE('',#10410,#10410,#9283,.T.);
#12702=EDGE_CURVE('',#10411,#10412,#5338,.T.);
#12703=EDGE_CURVE('',#10412,#10413,#9284,.T.);
#12704=EDGE_CURVE('',#10413,#10414,#9285,.T.);
#12705=EDGE_CURVE('',#10414,#10415,#9286,.T.);
#12706=EDGE_CURVE('',#10415,#10416,#9287,.T.);
#12707=EDGE_CURVE('',#10416,#10417,#9288,.T.);
#12708=EDGE_CURVE('',#10417,#10412,#9289,.T.);
#12709=EDGE_CURVE('',#10418,#10419,#5339,.T.);
#12710=EDGE_CURVE('',#10419,#10420,#9290,.T.);
#12711=EDGE_CURVE('',#10420,#10421,#9291,.T.);
#12712=EDGE_CURVE('',#10421,#10422,#9292,.T.);
#12713=EDGE_CURVE('',#10422,#10423,#9293,.T.);
#12714=EDGE_CURVE('',#10423,#10424,#9294,.T.);
#12715=EDGE_CURVE('',#10424,#10419,#9295,.T.);
#12716=EDGE_CURVE('',#10425,#10426,#5340,.T.);
#12717=EDGE_CURVE('',#10426,#10427,#9296,.T.);
#12718=EDGE_CURVE('',#10427,#10428,#9297,.T.);
#12719=EDGE_CURVE('',#10428,#10429,#9298,.T.);
#12720=EDGE_CURVE('',#10429,#10430,#9299,.T.);
#12721=EDGE_CURVE('',#10430,#10431,#9300,.T.);
#12722=EDGE_CURVE('',#10431,#10426,#9301,.T.);
#12723=EDGE_CURVE('',#10432,#10433,#5341,.T.);
#12724=EDGE_CURVE('',#10433,#10434,#9302,.T.);
#12725=EDGE_CURVE('',#10434,#10435,#9303,.T.);
#12726=EDGE_CURVE('',#10435,#10436,#9304,.T.);
#12727=EDGE_CURVE('',#10436,#10437,#9305,.T.);
#12728=EDGE_CURVE('',#10437,#10438,#9306,.T.);
#12729=EDGE_CURVE('',#10438,#10433,#9307,.T.);
#12730=EDGE_CURVE('',#10439,#10439,#9308,.T.);
#12731=EDGE_CURVE('',#10439,#10440,#5342,.T.);
#12732=EDGE_CURVE('',#10440,#10440,#9309,.T.);
#12733=EDGE_CURVE('',#10441,#10441,#9310,.T.);
#12734=EDGE_CURVE('',#10441,#10442,#5343,.T.);
#12735=EDGE_CURVE('',#10442,#10442,#9311,.T.);
#12736=EDGE_CURVE('',#10443,#10443,#9312,.T.);
#12737=EDGE_CURVE('',#10443,#10444,#5344,.T.);
#12738=EDGE_CURVE('',#10444,#10444,#9313,.T.);
#12739=EDGE_CURVE('',#10445,#10445,#9314,.T.);
#12740=EDGE_CURVE('',#10445,#10446,#5345,.T.);
#12741=EDGE_CURVE('',#10446,#10446,#9315,.T.);
#12742=EDGE_CURVE('',#10447,#10447,#9316,.T.);
#12743=EDGE_CURVE('',#10447,#10448,#5346,.T.);
#12744=EDGE_CURVE('',#10448,#10448,#9317,.T.);
#12745=EDGE_CURVE('',#10449,#10449,#9318,.T.);
#12746=EDGE_CURVE('',#10449,#10450,#5347,.T.);
#12747=EDGE_CURVE('',#10450,#10450,#9319,.T.);
#12748=EDGE_CURVE('',#10451,#10451,#9320,.T.);
#12749=EDGE_CURVE('',#10451,#10452,#5348,.T.);
#12750=EDGE_CURVE('',#10452,#10452,#9321,.T.);
#12751=EDGE_CURVE('',#10453,#10453,#9322,.T.);
#12752=EDGE_CURVE('',#10453,#10454,#5349,.T.);
#12753=EDGE_CURVE('',#10454,#10454,#9323,.T.);
#12754=EDGE_CURVE('',#10455,#10456,#5350,.T.);
#12755=EDGE_CURVE('',#10456,#10457,#5351,.T.);
#12756=EDGE_CURVE('',#10457,#10458,#5352,.T.);
#12757=EDGE_CURVE('',#10458,#10459,#5353,.T.);
#12758=EDGE_CURVE('',#10459,#10460,#5354,.T.);
#12759=EDGE_CURVE('',#10460,#10461,#5355,.T.);
#12760=EDGE_CURVE('',#10461,#10462,#5356,.T.);
#12761=EDGE_CURVE('',#10462,#10463,#5357,.T.);
#12762=EDGE_CURVE('',#10463,#10464,#5358,.T.);
#12763=EDGE_CURVE('',#10464,#10465,#5359,.T.);
#12764=EDGE_CURVE('',#10465,#10466,#5360,.T.);
#12765=EDGE_CURVE('',#10466,#10455,#5361,.T.);
#12766=EDGE_CURVE('',#10467,#10468,#5362,.T.);
#12767=EDGE_CURVE('',#10469,#10467,#5363,.T.);
#12768=EDGE_CURVE('',#10470,#10469,#5364,.T.);
#12769=EDGE_CURVE('',#10471,#10470,#5365,.T.);
#12770=EDGE_CURVE('',#10472,#10471,#5366,.T.);
#12771=EDGE_CURVE('',#10473,#10472,#5367,.T.);
#12772=EDGE_CURVE('',#10474,#10473,#5368,.T.);
#12773=EDGE_CURVE('',#10468,#10474,#5369,.T.);
#12774=EDGE_CURVE('',#10475,#10476,#5370,.T.);
#12775=EDGE_CURVE('',#10456,#10476,#5371,.T.);
#12776=EDGE_CURVE('',#10455,#10475,#5372,.T.);
#12777=EDGE_CURVE('',#10476,#10477,#5373,.T.);
#12778=EDGE_CURVE('',#10457,#10477,#5374,.T.);
#12779=EDGE_CURVE('',#10477,#10478,#5375,.T.);
#12780=EDGE_CURVE('',#10458,#10478,#5376,.T.);
#12781=EDGE_CURVE('',#10478,#10479,#5377,.T.);
#12782=EDGE_CURVE('',#10459,#10479,#5378,.T.);
#12783=EDGE_CURVE('',#10479,#10480,#5379,.T.);
#12784=EDGE_CURVE('',#10460,#10480,#5380,.T.);
#12785=EDGE_CURVE('',#10480,#10481,#5381,.T.);
#12786=EDGE_CURVE('',#10461,#10481,#5382,.T.);
#12787=EDGE_CURVE('',#10481,#10482,#5383,.T.);
#12788=EDGE_CURVE('',#10462,#10482,#5384,.T.);
#12789=EDGE_CURVE('',#10482,#10483,#5385,.T.);
#12790=EDGE_CURVE('',#10463,#10483,#5386,.T.);
#12791=EDGE_CURVE('',#10483,#10484,#5387,.T.);
#12792=EDGE_CURVE('',#10464,#10484,#5388,.T.);
#12793=EDGE_CURVE('',#10484,#10485,#5389,.T.);
#12794=EDGE_CURVE('',#10465,#10485,#5390,.T.);
#12795=EDGE_CURVE('',#10485,#10486,#5391,.T.);
#12796=EDGE_CURVE('',#10466,#10486,#5392,.T.);
#12797=EDGE_CURVE('',#10486,#10475,#5393,.T.);
#12798=EDGE_CURVE('',#10487,#10488,#5394,.T.);
#12799=EDGE_CURVE('',#10488,#10489,#5395,.T.);
#12800=EDGE_CURVE('',#10489,#10490,#5396,.T.);
#12801=EDGE_CURVE('',#10490,#10491,#5397,.T.);
#12802=EDGE_CURVE('',#10491,#10492,#5398,.T.);
#12803=EDGE_CURVE('',#10492,#10493,#5399,.T.);
#12804=EDGE_CURVE('',#10493,#10494,#5400,.T.);
#12805=EDGE_CURVE('',#10494,#10487,#5401,.T.);
#12806=EDGE_CURVE('',#10488,#10467,#5402,.T.);
#12807=EDGE_CURVE('',#10487,#10469,#5403,.T.);
#12808=EDGE_CURVE('',#10489,#10468,#5404,.T.);
#12809=EDGE_CURVE('',#10490,#10474,#5405,.T.);
#12810=EDGE_CURVE('',#10491,#10473,#5406,.T.);
#12811=EDGE_CURVE('',#10492,#10472,#5407,.T.);
#12812=EDGE_CURVE('',#10493,#10471,#5408,.T.);
#12813=EDGE_CURVE('',#10494,#10470,#5409,.T.);
#12814=EDGE_CURVE('',#10495,#10496,#5410,.T.);
#12815=EDGE_CURVE('',#10497,#10495,#5411,.T.);
#12816=EDGE_CURVE('',#10498,#10497,#5412,.T.);
#12817=EDGE_CURVE('',#10499,#10498,#5413,.T.);
#12818=EDGE_CURVE('',#10500,#10499,#5414,.T.);
#12819=EDGE_CURVE('',#10496,#10500,#5415,.T.);
#12820=EDGE_CURVE('',#10501,#10502,#5416,.T.);
#12821=EDGE_CURVE('',#10503,#10501,#5417,.T.);
#12822=EDGE_CURVE('',#10504,#10503,#5418,.T.);
#12823=EDGE_CURVE('',#10505,#10504,#5419,.T.);
#12824=EDGE_CURVE('',#10506,#10505,#5420,.T.);
#12825=EDGE_CURVE('',#10502,#10506,#5421,.T.);
#12826=EDGE_CURVE('',#10507,#10508,#5422,.T.);
#12827=EDGE_CURVE('',#10509,#10507,#5423,.T.);
#12828=EDGE_CURVE('',#10510,#10509,#5424,.T.);
#12829=EDGE_CURVE('',#10511,#10510,#5425,.T.);
#12830=EDGE_CURVE('',#10512,#10511,#5426,.T.);
#12831=EDGE_CURVE('',#10508,#10512,#5427,.T.);
#12832=EDGE_CURVE('',#10513,#10514,#5428,.T.);
#12833=EDGE_CURVE('',#10515,#10513,#5429,.T.);
#12834=EDGE_CURVE('',#10516,#10515,#5430,.T.);
#12835=EDGE_CURVE('',#10517,#10516,#5431,.T.);
#12836=EDGE_CURVE('',#10518,#10517,#5432,.T.);
#12837=EDGE_CURVE('',#10514,#10518,#5433,.T.);
#12838=EDGE_CURVE('',#10519,#10499,#5434,.T.);
#12839=EDGE_CURVE('',#10434,#10519,#5435,.T.);
#12840=EDGE_CURVE('',#10520,#10434,#5436,.T.);
#12841=EDGE_CURVE('',#10520,#10500,#5437,.T.);
#12842=EDGE_CURVE('',#10433,#10520,#5438,.T.);
#12843=EDGE_CURVE('',#10521,#10433,#5439,.T.);
#12844=EDGE_CURVE('',#10521,#10496,#5440,.T.);
#12845=EDGE_CURVE('',#10438,#10521,#5441,.T.);
#12846=EDGE_CURVE('',#10522,#10438,#5442,.T.);
#12847=EDGE_CURVE('',#10522,#10495,#5443,.T.);
#12848=EDGE_CURVE('',#10437,#10522,#5444,.T.);
#12849=EDGE_CURVE('',#10523,#10437,#5445,.T.);
#12850=EDGE_CURVE('',#10523,#10497,#5446,.T.);
#12851=EDGE_CURVE('',#10436,#10523,#5447,.T.);
#12852=EDGE_CURVE('',#10524,#10436,#5448,.T.);
#12853=EDGE_CURVE('',#10524,#10498,#5449,.T.);
#12854=EDGE_CURVE('',#10435,#10524,#5450,.T.);
#12855=EDGE_CURVE('',#10519,#10435,#5451,.T.);
#12856=EDGE_CURVE('',#10525,#10505,#5452,.T.);
#12857=EDGE_CURVE('',#10428,#10525,#5453,.T.);
#12858=EDGE_CURVE('',#10526,#10428,#5454,.T.);
#12859=EDGE_CURVE('',#10526,#10506,#5455,.T.);
#12860=EDGE_CURVE('',#10427,#10526,#5456,.T.);
#12861=EDGE_CURVE('',#10527,#10427,#5457,.T.);
#12862=EDGE_CURVE('',#10527,#10502,#5458,.T.);
#12863=EDGE_CURVE('',#10426,#10527,#5459,.T.);
#12864=EDGE_CURVE('',#10528,#10426,#5460,.T.);
#12865=EDGE_CURVE('',#10528,#10501,#5461,.T.);
#12866=EDGE_CURVE('',#10431,#10528,#5462,.T.);
#12867=EDGE_CURVE('',#10529,#10431,#5463,.T.);
#12868=EDGE_CURVE('',#10529,#10503,#5464,.T.);
#12869=EDGE_CURVE('',#10430,#10529,#5465,.T.);
#12870=EDGE_CURVE('',#10530,#10430,#5466,.T.);
#12871=EDGE_CURVE('',#10530,#10504,#5467,.T.);
#12872=EDGE_CURVE('',#10429,#10530,#5468,.T.);
#12873=EDGE_CURVE('',#10525,#10429,#5469,.T.);
#12874=EDGE_CURVE('',#10531,#10517,#5470,.T.);
#12875=EDGE_CURVE('',#10421,#10531,#5471,.T.);
#12876=EDGE_CURVE('',#10532,#10421,#5472,.T.);
#12877=EDGE_CURVE('',#10532,#10518,#5473,.T.);
#12878=EDGE_CURVE('',#10420,#10532,#5474,.T.);
#12879=EDGE_CURVE('',#10533,#10420,#5475,.T.);
#12880=EDGE_CURVE('',#10533,#10514,#5476,.T.);
#12881=EDGE_CURVE('',#10419,#10533,#5477,.T.);
#12882=EDGE_CURVE('',#10534,#10419,#5478,.T.);
#12883=EDGE_CURVE('',#10534,#10513,#5479,.T.);
#12884=EDGE_CURVE('',#10424,#10534,#5480,.T.);
#12885=EDGE_CURVE('',#10535,#10424,#5481,.T.);
#12886=EDGE_CURVE('',#10535,#10515,#5482,.T.);
#12887=EDGE_CURVE('',#10423,#10535,#5483,.T.);
#12888=EDGE_CURVE('',#10536,#10423,#5484,.T.);
#12889=EDGE_CURVE('',#10536,#10516,#5485,.T.);
#12890=EDGE_CURVE('',#10422,#10536,#5486,.T.);
#12891=EDGE_CURVE('',#10531,#10422,#5487,.T.);
#12892=EDGE_CURVE('',#10537,#10511,#5488,.T.);
#12893=EDGE_CURVE('',#10414,#10537,#5489,.T.);
#12894=EDGE_CURVE('',#10538,#10414,#5490,.T.);
#12895=EDGE_CURVE('',#10538,#10512,#5491,.T.);
#12896=EDGE_CURVE('',#10413,#10538,#5492,.T.);
#12897=EDGE_CURVE('',#10539,#10413,#5493,.T.);
#12898=EDGE_CURVE('',#10539,#10508,#5494,.T.);
#12899=EDGE_CURVE('',#10412,#10539,#5495,.T.);
#12900=EDGE_CURVE('',#10540,#10412,#5496,.T.);
#12901=EDGE_CURVE('',#10540,#10507,#5497,.T.);
#12902=EDGE_CURVE('',#10417,#10540,#5498,.T.);
#12903=EDGE_CURVE('',#10541,#10417,#5499,.T.);
#12904=EDGE_CURVE('',#10541,#10509,#5500,.T.);
#12905=EDGE_CURVE('',#10416,#10541,#5501,.T.);
#12906=EDGE_CURVE('',#10542,#10416,#5502,.T.);
#12907=EDGE_CURVE('',#10542,#10510,#5503,.T.);
#12908=EDGE_CURVE('',#10415,#10542,#5504,.T.);
#12909=EDGE_CURVE('',#10537,#10415,#5505,.T.);
#16272=ORIENTED_EDGE('',*,*,#12681,.F.);
#16273=ORIENTED_EDGE('',*,*,#12682,.T.);
#16274=ORIENTED_EDGE('',*,*,#12683,.T.);
#16275=ORIENTED_EDGE('',*,*,#12682,.F.);
#16276=ORIENTED_EDGE('',*,*,#12684,.F.);
#16277=ORIENTED_EDGE('',*,*,#12685,.T.);
#16278=ORIENTED_EDGE('',*,*,#12686,.T.);
#16279=ORIENTED_EDGE('',*,*,#12685,.F.);
#16280=ORIENTED_EDGE('',*,*,#12687,.F.);
#16281=ORIENTED_EDGE('',*,*,#12688,.T.);
#16282=ORIENTED_EDGE('',*,*,#12689,.T.);
#16283=ORIENTED_EDGE('',*,*,#12688,.F.);
#16284=ORIENTED_EDGE('',*,*,#12690,.F.);
#16285=ORIENTED_EDGE('',*,*,#12691,.T.);
#16286=ORIENTED_EDGE('',*,*,#12692,.T.);
#16287=ORIENTED_EDGE('',*,*,#12691,.F.);
#16288=ORIENTED_EDGE('',*,*,#12693,.F.);
#16289=ORIENTED_EDGE('',*,*,#12694,.T.);
#16290=ORIENTED_EDGE('',*,*,#12695,.T.);
#16291=ORIENTED_EDGE('',*,*,#12694,.F.);
#16292=ORIENTED_EDGE('',*,*,#12696,.F.);
#16293=ORIENTED_EDGE('',*,*,#12697,.T.);
#16294=ORIENTED_EDGE('',*,*,#12698,.T.);
#16295=ORIENTED_EDGE('',*,*,#12697,.F.);
#16296=ORIENTED_EDGE('',*,*,#12699,.F.);
#16297=ORIENTED_EDGE('',*,*,#12700,.T.);
#16298=ORIENTED_EDGE('',*,*,#12701,.T.);
#16299=ORIENTED_EDGE('',*,*,#12700,.F.);
#16300=ORIENTED_EDGE('',*,*,#12702,.T.);
#16301=ORIENTED_EDGE('',*,*,#12703,.T.);
#16302=ORIENTED_EDGE('',*,*,#12704,.T.);
#16303=ORIENTED_EDGE('',*,*,#12705,.T.);
#16304=ORIENTED_EDGE('',*,*,#12706,.T.);
#16305=ORIENTED_EDGE('',*,*,#12707,.T.);
#16306=ORIENTED_EDGE('',*,*,#12708,.T.);
#16307=ORIENTED_EDGE('',*,*,#12702,.F.);
#16308=ORIENTED_EDGE('',*,*,#12709,.T.);
#16309=ORIENTED_EDGE('',*,*,#12710,.T.);
#16310=ORIENTED_EDGE('',*,*,#12711,.T.);
#16311=ORIENTED_EDGE('',*,*,#12712,.T.);
#16312=ORIENTED_EDGE('',*,*,#12713,.T.);
#16313=ORIENTED_EDGE('',*,*,#12714,.T.);
#16314=ORIENTED_EDGE('',*,*,#12715,.T.);
#16315=ORIENTED_EDGE('',*,*,#12709,.F.);
#16316=ORIENTED_EDGE('',*,*,#12716,.T.);
#16317=ORIENTED_EDGE('',*,*,#12717,.T.);
#16318=ORIENTED_EDGE('',*,*,#12718,.T.);
#16319=ORIENTED_EDGE('',*,*,#12719,.T.);
#16320=ORIENTED_EDGE('',*,*,#12720,.T.);
#16321=ORIENTED_EDGE('',*,*,#12721,.T.);
#16322=ORIENTED_EDGE('',*,*,#12722,.T.);
#16323=ORIENTED_EDGE('',*,*,#12716,.F.);
#16324=ORIENTED_EDGE('',*,*,#12723,.T.);
#16325=ORIENTED_EDGE('',*,*,#12724,.T.);
#16326=ORIENTED_EDGE('',*,*,#12725,.T.);
#16327=ORIENTED_EDGE('',*,*,#12726,.T.);
#16328=ORIENTED_EDGE('',*,*,#12727,.T.);
#16329=ORIENTED_EDGE('',*,*,#12728,.T.);
#16330=ORIENTED_EDGE('',*,*,#12729,.T.);
#16331=ORIENTED_EDGE('',*,*,#12723,.F.);
#16332=ORIENTED_EDGE('',*,*,#12730,.T.);
#16333=ORIENTED_EDGE('',*,*,#12731,.T.);
#16334=ORIENTED_EDGE('',*,*,#12732,.F.);
#16335=ORIENTED_EDGE('',*,*,#12731,.F.);
#16336=ORIENTED_EDGE('',*,*,#12733,.T.);
#16337=ORIENTED_EDGE('',*,*,#12734,.T.);
#16338=ORIENTED_EDGE('',*,*,#12735,.F.);
#16339=ORIENTED_EDGE('',*,*,#12734,.F.);
#16340=ORIENTED_EDGE('',*,*,#12736,.T.);
#16341=ORIENTED_EDGE('',*,*,#12737,.T.);
#16342=ORIENTED_EDGE('',*,*,#12738,.F.);
#16343=ORIENTED_EDGE('',*,*,#12737,.F.);
#16344=ORIENTED_EDGE('',*,*,#12739,.T.);
#16345=ORIENTED_EDGE('',*,*,#12740,.T.);
#16346=ORIENTED_EDGE('',*,*,#12741,.F.);
#16347=ORIENTED_EDGE('',*,*,#12740,.F.);
#16348=ORIENTED_EDGE('',*,*,#12742,.T.);
#16349=ORIENTED_EDGE('',*,*,#12743,.T.);
#16350=ORIENTED_EDGE('',*,*,#12744,.T.);
#16351=ORIENTED_EDGE('',*,*,#12743,.F.);
#16352=ORIENTED_EDGE('',*,*,#12745,.T.);
#16353=ORIENTED_EDGE('',*,*,#12746,.T.);
#16354=ORIENTED_EDGE('',*,*,#12747,.T.);
#16355=ORIENTED_EDGE('',*,*,#12746,.F.);
#16356=ORIENTED_EDGE('',*,*,#12748,.T.);
#16357=ORIENTED_EDGE('',*,*,#12749,.T.);
#16358=ORIENTED_EDGE('',*,*,#12750,.T.);
#16359=ORIENTED_EDGE('',*,*,#12749,.F.);
#16360=ORIENTED_EDGE('',*,*,#12751,.T.);
#16361=ORIENTED_EDGE('',*,*,#12752,.T.);
#16362=ORIENTED_EDGE('',*,*,#12753,.T.);
#16363=ORIENTED_EDGE('',*,*,#12752,.F.);
#16364=ORIENTED_EDGE('',*,*,#12747,.F.);
#16365=ORIENTED_EDGE('',*,*,#12730,.F.);
#16366=ORIENTED_EDGE('',*,*,#12744,.F.);
#16367=ORIENTED_EDGE('',*,*,#12733,.F.);
#16368=ORIENTED_EDGE('',*,*,#12750,.F.);
#16369=ORIENTED_EDGE('',*,*,#12736,.F.);
#16370=ORIENTED_EDGE('',*,*,#12753,.F.);
#16371=ORIENTED_EDGE('',*,*,#12739,.F.);
#16372=ORIENTED_EDGE('',*,*,#12754,.T.);
#16373=ORIENTED_EDGE('',*,*,#12755,.T.);
#16374=ORIENTED_EDGE('',*,*,#12756,.T.);
#16375=ORIENTED_EDGE('',*,*,#12757,.T.);
#16376=ORIENTED_EDGE('',*,*,#12758,.T.);
#16377=ORIENTED_EDGE('',*,*,#12759,.T.);
#16378=ORIENTED_EDGE('',*,*,#12760,.T.);
#16379=ORIENTED_EDGE('',*,*,#12761,.T.);
#16380=ORIENTED_EDGE('',*,*,#12762,.T.);
#16381=ORIENTED_EDGE('',*,*,#12763,.T.);
#16382=ORIENTED_EDGE('',*,*,#12764,.T.);
#16383=ORIENTED_EDGE('',*,*,#12765,.T.);
#16384=ORIENTED_EDGE('',*,*,#12766,.F.);
#16385=ORIENTED_EDGE('',*,*,#12767,.F.);
#16386=ORIENTED_EDGE('',*,*,#12768,.F.);
#16387=ORIENTED_EDGE('',*,*,#12769,.F.);
#16388=ORIENTED_EDGE('',*,*,#12770,.F.);
#16389=ORIENTED_EDGE('',*,*,#12771,.F.);
#16390=ORIENTED_EDGE('',*,*,#12772,.F.);
#16391=ORIENTED_EDGE('',*,*,#12773,.F.);
#16392=ORIENTED_EDGE('',*,*,#12774,.T.);
#16393=ORIENTED_EDGE('',*,*,#12775,.F.);
#16394=ORIENTED_EDGE('',*,*,#12754,.F.);
#16395=ORIENTED_EDGE('',*,*,#12776,.T.);
#16396=ORIENTED_EDGE('',*,*,#12683,.F.);
#16397=ORIENTED_EDGE('',*,*,#12777,.T.);
#16398=ORIENTED_EDGE('',*,*,#12778,.F.);
#16399=ORIENTED_EDGE('',*,*,#12755,.F.);
#16400=ORIENTED_EDGE('',*,*,#12775,.T.);
#16401=ORIENTED_EDGE('',*,*,#12779,.T.);
#16402=ORIENTED_EDGE('',*,*,#12780,.F.);
#16403=ORIENTED_EDGE('',*,*,#12756,.F.);
#16404=ORIENTED_EDGE('',*,*,#12778,.T.);
#16405=ORIENTED_EDGE('',*,*,#12781,.T.);
#16406=ORIENTED_EDGE('',*,*,#12782,.F.);
#16407=ORIENTED_EDGE('',*,*,#12757,.F.);
#16408=ORIENTED_EDGE('',*,*,#12780,.T.);
#16409=ORIENTED_EDGE('',*,*,#12681,.T.);
#16410=ORIENTED_EDGE('',*,*,#12684,.T.);
#16411=ORIENTED_EDGE('',*,*,#12783,.T.);
#16412=ORIENTED_EDGE('',*,*,#12784,.F.);
#16413=ORIENTED_EDGE('',*,*,#12758,.F.);
#16414=ORIENTED_EDGE('',*,*,#12782,.T.);
#16415=ORIENTED_EDGE('',*,*,#12785,.T.);
#16416=ORIENTED_EDGE('',*,*,#12786,.F.);
#16417=ORIENTED_EDGE('',*,*,#12759,.F.);
#16418=ORIENTED_EDGE('',*,*,#12784,.T.);
#16419=ORIENTED_EDGE('',*,*,#12787,.T.);
#16420=ORIENTED_EDGE('',*,*,#12788,.F.);
#16421=ORIENTED_EDGE('',*,*,#12760,.F.);
#16422=ORIENTED_EDGE('',*,*,#12786,.T.);
#16423=ORIENTED_EDGE('',*,*,#12686,.F.);
#16424=ORIENTED_EDGE('',*,*,#12789,.T.);
#16425=ORIENTED_EDGE('',*,*,#12790,.F.);
#16426=ORIENTED_EDGE('',*,*,#12761,.F.);
#16427=ORIENTED_EDGE('',*,*,#12788,.T.);
#16428=ORIENTED_EDGE('',*,*,#12791,.T.);
#16429=ORIENTED_EDGE('',*,*,#12792,.F.);
#16430=ORIENTED_EDGE('',*,*,#12762,.F.);
#16431=ORIENTED_EDGE('',*,*,#12790,.T.);
#16432=ORIENTED_EDGE('',*,*,#12793,.T.);
#16433=ORIENTED_EDGE('',*,*,#12794,.F.);
#16434=ORIENTED_EDGE('',*,*,#12763,.F.);
#16435=ORIENTED_EDGE('',*,*,#12792,.T.);
#16436=ORIENTED_EDGE('',*,*,#12795,.T.);
#16437=ORIENTED_EDGE('',*,*,#12796,.F.);
#16438=ORIENTED_EDGE('',*,*,#12764,.F.);
#16439=ORIENTED_EDGE('',*,*,#12794,.T.);
#16440=ORIENTED_EDGE('',*,*,#12797,.T.);
#16441=ORIENTED_EDGE('',*,*,#12776,.F.);
#16442=ORIENTED_EDGE('',*,*,#12765,.F.);
#16443=ORIENTED_EDGE('',*,*,#12796,.T.);
#16444=ORIENTED_EDGE('',*,*,#12774,.F.);
#16445=ORIENTED_EDGE('',*,*,#12797,.F.);
#16446=ORIENTED_EDGE('',*,*,#12795,.F.);
#16447=ORIENTED_EDGE('',*,*,#12793,.F.);
#16448=ORIENTED_EDGE('',*,*,#12791,.F.);
#16449=ORIENTED_EDGE('',*,*,#12789,.F.);
#16450=ORIENTED_EDGE('',*,*,#12787,.F.);
#16451=ORIENTED_EDGE('',*,*,#12785,.F.);
#16452=ORIENTED_EDGE('',*,*,#12783,.F.);
#16453=ORIENTED_EDGE('',*,*,#12781,.F.);
#16454=ORIENTED_EDGE('',*,*,#12779,.F.);
#16455=ORIENTED_EDGE('',*,*,#12777,.F.);
#16456=ORIENTED_EDGE('',*,*,#12699,.T.);
#16457=ORIENTED_EDGE('',*,*,#12798,.T.);
#16458=ORIENTED_EDGE('',*,*,#12799,.T.);
#16459=ORIENTED_EDGE('',*,*,#12800,.T.);
#16460=ORIENTED_EDGE('',*,*,#12801,.T.);
#16461=ORIENTED_EDGE('',*,*,#12802,.T.);
#16462=ORIENTED_EDGE('',*,*,#12803,.T.);
#16463=ORIENTED_EDGE('',*,*,#12804,.T.);
#16464=ORIENTED_EDGE('',*,*,#12805,.T.);
#16465=ORIENTED_EDGE('',*,*,#12751,.F.);
#16466=ORIENTED_EDGE('',*,*,#12748,.F.);
#16467=ORIENTED_EDGE('',*,*,#12745,.F.);
#16468=ORIENTED_EDGE('',*,*,#12742,.F.);
#16469=ORIENTED_EDGE('',*,*,#12689,.F.);
#16470=ORIENTED_EDGE('',*,*,#12767,.T.);
#16471=ORIENTED_EDGE('',*,*,#12806,.F.);
#16472=ORIENTED_EDGE('',*,*,#12798,.F.);
#16473=ORIENTED_EDGE('',*,*,#12807,.T.);
#16474=ORIENTED_EDGE('',*,*,#12766,.T.);
#16475=ORIENTED_EDGE('',*,*,#12808,.F.);
#16476=ORIENTED_EDGE('',*,*,#12799,.F.);
#16477=ORIENTED_EDGE('',*,*,#12806,.T.);
#16478=ORIENTED_EDGE('',*,*,#12773,.T.);
#16479=ORIENTED_EDGE('',*,*,#12809,.F.);
#16480=ORIENTED_EDGE('',*,*,#12800,.F.);
#16481=ORIENTED_EDGE('',*,*,#12808,.T.);
#16482=ORIENTED_EDGE('',*,*,#12772,.T.);
#16483=ORIENTED_EDGE('',*,*,#12810,.F.);
#16484=ORIENTED_EDGE('',*,*,#12801,.F.);
#16485=ORIENTED_EDGE('',*,*,#12809,.T.);
#16486=ORIENTED_EDGE('',*,*,#12771,.T.);
#16487=ORIENTED_EDGE('',*,*,#12811,.F.);
#16488=ORIENTED_EDGE('',*,*,#12802,.F.);
#16489=ORIENTED_EDGE('',*,*,#12810,.T.);
#16490=ORIENTED_EDGE('',*,*,#12770,.T.);
#16491=ORIENTED_EDGE('',*,*,#12812,.F.);
#16492=ORIENTED_EDGE('',*,*,#12803,.F.);
#16493=ORIENTED_EDGE('',*,*,#12811,.T.);
#16494=ORIENTED_EDGE('',*,*,#12769,.T.);
#16495=ORIENTED_EDGE('',*,*,#12813,.F.);
#16496=ORIENTED_EDGE('',*,*,#12804,.F.);
#16497=ORIENTED_EDGE('',*,*,#12812,.T.);
#16498=ORIENTED_EDGE('',*,*,#12768,.T.);
#16499=ORIENTED_EDGE('',*,*,#12807,.F.);
#16500=ORIENTED_EDGE('',*,*,#12805,.F.);
#16501=ORIENTED_EDGE('',*,*,#12813,.T.);
#16502=ORIENTED_EDGE('',*,*,#12741,.T.);
#16503=ORIENTED_EDGE('',*,*,#12814,.F.);
#16504=ORIENTED_EDGE('',*,*,#12815,.F.);
#16505=ORIENTED_EDGE('',*,*,#12816,.F.);
#16506=ORIENTED_EDGE('',*,*,#12817,.F.);
#16507=ORIENTED_EDGE('',*,*,#12818,.F.);
#16508=ORIENTED_EDGE('',*,*,#12819,.F.);
#16509=ORIENTED_EDGE('',*,*,#12738,.T.);
#16510=ORIENTED_EDGE('',*,*,#12820,.F.);
#16511=ORIENTED_EDGE('',*,*,#12821,.F.);
#16512=ORIENTED_EDGE('',*,*,#12822,.F.);
#16513=ORIENTED_EDGE('',*,*,#12823,.F.);
#16514=ORIENTED_EDGE('',*,*,#12824,.F.);
#16515=ORIENTED_EDGE('',*,*,#12825,.F.);
#16516=ORIENTED_EDGE('',*,*,#12735,.T.);
#16517=ORIENTED_EDGE('',*,*,#12826,.F.);
#16518=ORIENTED_EDGE('',*,*,#12827,.F.);
#16519=ORIENTED_EDGE('',*,*,#12828,.F.);
#16520=ORIENTED_EDGE('',*,*,#12829,.F.);
#16521=ORIENTED_EDGE('',*,*,#12830,.F.);
#16522=ORIENTED_EDGE('',*,*,#12831,.F.);
#16523=ORIENTED_EDGE('',*,*,#12732,.T.);
#16524=ORIENTED_EDGE('',*,*,#12832,.F.);
#16525=ORIENTED_EDGE('',*,*,#12833,.F.);
#16526=ORIENTED_EDGE('',*,*,#12834,.F.);
#16527=ORIENTED_EDGE('',*,*,#12835,.F.);
#16528=ORIENTED_EDGE('',*,*,#12836,.F.);
#16529=ORIENTED_EDGE('',*,*,#12837,.F.);
#16530=ORIENTED_EDGE('',*,*,#12818,.T.);
#16531=ORIENTED_EDGE('',*,*,#12838,.F.);
#16532=ORIENTED_EDGE('',*,*,#12839,.F.);
#16533=ORIENTED_EDGE('',*,*,#12840,.F.);
#16534=ORIENTED_EDGE('',*,*,#12841,.T.);
#16535=ORIENTED_EDGE('',*,*,#12819,.T.);
#16536=ORIENTED_EDGE('',*,*,#12841,.F.);
#16537=ORIENTED_EDGE('',*,*,#12842,.F.);
#16538=ORIENTED_EDGE('',*,*,#12843,.F.);
#16539=ORIENTED_EDGE('',*,*,#12844,.T.);
#16540=ORIENTED_EDGE('',*,*,#12814,.T.);
#16541=ORIENTED_EDGE('',*,*,#12844,.F.);
#16542=ORIENTED_EDGE('',*,*,#12845,.F.);
#16543=ORIENTED_EDGE('',*,*,#12846,.F.);
#16544=ORIENTED_EDGE('',*,*,#12847,.T.);
#16545=ORIENTED_EDGE('',*,*,#12815,.T.);
#16546=ORIENTED_EDGE('',*,*,#12847,.F.);
#16547=ORIENTED_EDGE('',*,*,#12848,.F.);
#16548=ORIENTED_EDGE('',*,*,#12849,.F.);
#16549=ORIENTED_EDGE('',*,*,#12850,.T.);
#16550=ORIENTED_EDGE('',*,*,#12816,.T.);
#16551=ORIENTED_EDGE('',*,*,#12850,.F.);
#16552=ORIENTED_EDGE('',*,*,#12851,.F.);
#16553=ORIENTED_EDGE('',*,*,#12852,.F.);
#16554=ORIENTED_EDGE('',*,*,#12853,.T.);
#16555=ORIENTED_EDGE('',*,*,#12817,.T.);
#16556=ORIENTED_EDGE('',*,*,#12853,.F.);
#16557=ORIENTED_EDGE('',*,*,#12854,.F.);
#16558=ORIENTED_EDGE('',*,*,#12855,.F.);
#16559=ORIENTED_EDGE('',*,*,#12838,.T.);
#16560=ORIENTED_EDGE('',*,*,#12726,.F.);
#16561=ORIENTED_EDGE('',*,*,#12854,.T.);
#16562=ORIENTED_EDGE('',*,*,#12852,.T.);
#16563=ORIENTED_EDGE('',*,*,#12725,.F.);
#16564=ORIENTED_EDGE('',*,*,#12839,.T.);
#16565=ORIENTED_EDGE('',*,*,#12855,.T.);
#16566=ORIENTED_EDGE('',*,*,#12724,.F.);
#16567=ORIENTED_EDGE('',*,*,#12842,.T.);
#16568=ORIENTED_EDGE('',*,*,#12840,.T.);
#16569=ORIENTED_EDGE('',*,*,#12729,.F.);
#16570=ORIENTED_EDGE('',*,*,#12845,.T.);
#16571=ORIENTED_EDGE('',*,*,#12843,.T.);
#16572=ORIENTED_EDGE('',*,*,#12728,.F.);
#16573=ORIENTED_EDGE('',*,*,#12848,.T.);
#16574=ORIENTED_EDGE('',*,*,#12846,.T.);
#16575=ORIENTED_EDGE('',*,*,#12727,.F.);
#16576=ORIENTED_EDGE('',*,*,#12851,.T.);
#16577=ORIENTED_EDGE('',*,*,#12849,.T.);
#16578=ORIENTED_EDGE('',*,*,#12824,.T.);
#16579=ORIENTED_EDGE('',*,*,#12856,.F.);
#16580=ORIENTED_EDGE('',*,*,#12857,.F.);
#16581=ORIENTED_EDGE('',*,*,#12858,.F.);
#16582=ORIENTED_EDGE('',*,*,#12859,.T.);
#16583=ORIENTED_EDGE('',*,*,#12825,.T.);
#16584=ORIENTED_EDGE('',*,*,#12859,.F.);
#16585=ORIENTED_EDGE('',*,*,#12860,.F.);
#16586=ORIENTED_EDGE('',*,*,#12861,.F.);
#16587=ORIENTED_EDGE('',*,*,#12862,.T.);
#16588=ORIENTED_EDGE('',*,*,#12820,.T.);
#16589=ORIENTED_EDGE('',*,*,#12862,.F.);
#16590=ORIENTED_EDGE('',*,*,#12863,.F.);
#16591=ORIENTED_EDGE('',*,*,#12864,.F.);
#16592=ORIENTED_EDGE('',*,*,#12865,.T.);
#16593=ORIENTED_EDGE('',*,*,#12821,.T.);
#16594=ORIENTED_EDGE('',*,*,#12865,.F.);
#16595=ORIENTED_EDGE('',*,*,#12866,.F.);
#16596=ORIENTED_EDGE('',*,*,#12867,.F.);
#16597=ORIENTED_EDGE('',*,*,#12868,.T.);
#16598=ORIENTED_EDGE('',*,*,#12822,.T.);
#16599=ORIENTED_EDGE('',*,*,#12868,.F.);
#16600=ORIENTED_EDGE('',*,*,#12869,.F.);
#16601=ORIENTED_EDGE('',*,*,#12870,.F.);
#16602=ORIENTED_EDGE('',*,*,#12871,.T.);
#16603=ORIENTED_EDGE('',*,*,#12823,.T.);
#16604=ORIENTED_EDGE('',*,*,#12871,.F.);
#16605=ORIENTED_EDGE('',*,*,#12872,.F.);
#16606=ORIENTED_EDGE('',*,*,#12873,.F.);
#16607=ORIENTED_EDGE('',*,*,#12856,.T.);
#16608=ORIENTED_EDGE('',*,*,#12719,.F.);
#16609=ORIENTED_EDGE('',*,*,#12857,.T.);
#16610=ORIENTED_EDGE('',*,*,#12873,.T.);
#16611=ORIENTED_EDGE('',*,*,#12718,.F.);
#16612=ORIENTED_EDGE('',*,*,#12860,.T.);
#16613=ORIENTED_EDGE('',*,*,#12858,.T.);
#16614=ORIENTED_EDGE('',*,*,#12717,.F.);
#16615=ORIENTED_EDGE('',*,*,#12863,.T.);
#16616=ORIENTED_EDGE('',*,*,#12861,.T.);
#16617=ORIENTED_EDGE('',*,*,#12722,.F.);
#16618=ORIENTED_EDGE('',*,*,#12866,.T.);
#16619=ORIENTED_EDGE('',*,*,#12864,.T.);
#16620=ORIENTED_EDGE('',*,*,#12721,.F.);
#16621=ORIENTED_EDGE('',*,*,#12869,.T.);
#16622=ORIENTED_EDGE('',*,*,#12867,.T.);
#16623=ORIENTED_EDGE('',*,*,#12720,.F.);
#16624=ORIENTED_EDGE('',*,*,#12872,.T.);
#16625=ORIENTED_EDGE('',*,*,#12870,.T.);
#16626=ORIENTED_EDGE('',*,*,#12836,.T.);
#16627=ORIENTED_EDGE('',*,*,#12874,.F.);
#16628=ORIENTED_EDGE('',*,*,#12875,.F.);
#16629=ORIENTED_EDGE('',*,*,#12876,.F.);
#16630=ORIENTED_EDGE('',*,*,#12877,.T.);
#16631=ORIENTED_EDGE('',*,*,#12837,.T.);
#16632=ORIENTED_EDGE('',*,*,#12877,.F.);
#16633=ORIENTED_EDGE('',*,*,#12878,.F.);
#16634=ORIENTED_EDGE('',*,*,#12879,.F.);
#16635=ORIENTED_EDGE('',*,*,#12880,.T.);
#16636=ORIENTED_EDGE('',*,*,#12832,.T.);
#16637=ORIENTED_EDGE('',*,*,#12880,.F.);
#16638=ORIENTED_EDGE('',*,*,#12881,.F.);
#16639=ORIENTED_EDGE('',*,*,#12882,.F.);
#16640=ORIENTED_EDGE('',*,*,#12883,.T.);
#16641=ORIENTED_EDGE('',*,*,#12833,.T.);
#16642=ORIENTED_EDGE('',*,*,#12883,.F.);
#16643=ORIENTED_EDGE('',*,*,#12884,.F.);
#16644=ORIENTED_EDGE('',*,*,#12885,.F.);
#16645=ORIENTED_EDGE('',*,*,#12886,.T.);
#16646=ORIENTED_EDGE('',*,*,#12834,.T.);
#16647=ORIENTED_EDGE('',*,*,#12886,.F.);
#16648=ORIENTED_EDGE('',*,*,#12887,.F.);
#16649=ORIENTED_EDGE('',*,*,#12888,.F.);
#16650=ORIENTED_EDGE('',*,*,#12889,.T.);
#16651=ORIENTED_EDGE('',*,*,#12835,.T.);
#16652=ORIENTED_EDGE('',*,*,#12889,.F.);
#16653=ORIENTED_EDGE('',*,*,#12890,.F.);
#16654=ORIENTED_EDGE('',*,*,#12891,.F.);
#16655=ORIENTED_EDGE('',*,*,#12874,.T.);
#16656=ORIENTED_EDGE('',*,*,#12712,.F.);
#16657=ORIENTED_EDGE('',*,*,#12875,.T.);
#16658=ORIENTED_EDGE('',*,*,#12891,.T.);
#16659=ORIENTED_EDGE('',*,*,#12711,.F.);
#16660=ORIENTED_EDGE('',*,*,#12878,.T.);
#16661=ORIENTED_EDGE('',*,*,#12876,.T.);
#16662=ORIENTED_EDGE('',*,*,#12710,.F.);
#16663=ORIENTED_EDGE('',*,*,#12881,.T.);
#16664=ORIENTED_EDGE('',*,*,#12879,.T.);
#16665=ORIENTED_EDGE('',*,*,#12715,.F.);
#16666=ORIENTED_EDGE('',*,*,#12884,.T.);
#16667=ORIENTED_EDGE('',*,*,#12882,.T.);
#16668=ORIENTED_EDGE('',*,*,#12714,.F.);
#16669=ORIENTED_EDGE('',*,*,#12887,.T.);
#16670=ORIENTED_EDGE('',*,*,#12885,.T.);
#16671=ORIENTED_EDGE('',*,*,#12713,.F.);
#16672=ORIENTED_EDGE('',*,*,#12890,.T.);
#16673=ORIENTED_EDGE('',*,*,#12888,.T.);
#16674=ORIENTED_EDGE('',*,*,#12830,.T.);
#16675=ORIENTED_EDGE('',*,*,#12892,.F.);
#16676=ORIENTED_EDGE('',*,*,#12893,.F.);
#16677=ORIENTED_EDGE('',*,*,#12894,.F.);
#16678=ORIENTED_EDGE('',*,*,#12895,.T.);
#16679=ORIENTED_EDGE('',*,*,#12831,.T.);
#16680=ORIENTED_EDGE('',*,*,#12895,.F.);
#16681=ORIENTED_EDGE('',*,*,#12896,.F.);
#16682=ORIENTED_EDGE('',*,*,#12897,.F.);
#16683=ORIENTED_EDGE('',*,*,#12898,.T.);
#16684=ORIENTED_EDGE('',*,*,#12826,.T.);
#16685=ORIENTED_EDGE('',*,*,#12898,.F.);
#16686=ORIENTED_EDGE('',*,*,#12899,.F.);
#16687=ORIENTED_EDGE('',*,*,#12900,.F.);
#16688=ORIENTED_EDGE('',*,*,#12901,.T.);
#16689=ORIENTED_EDGE('',*,*,#12827,.T.);
#16690=ORIENTED_EDGE('',*,*,#12901,.F.);
#16691=ORIENTED_EDGE('',*,*,#12902,.F.);
#16692=ORIENTED_EDGE('',*,*,#12903,.F.);
#16693=ORIENTED_EDGE('',*,*,#12904,.T.);
#16694=ORIENTED_EDGE('',*,*,#12828,.T.);
#16695=ORIENTED_EDGE('',*,*,#12904,.F.);
#16696=ORIENTED_EDGE('',*,*,#12905,.F.);
#16697=ORIENTED_EDGE('',*,*,#12906,.F.);
#16698=ORIENTED_EDGE('',*,*,#12907,.T.);
#16699=ORIENTED_EDGE('',*,*,#12829,.T.);
#16700=ORIENTED_EDGE('',*,*,#12907,.F.);
#16701=ORIENTED_EDGE('',*,*,#12908,.F.);
#16702=ORIENTED_EDGE('',*,*,#12909,.F.);
#16703=ORIENTED_EDGE('',*,*,#12892,.T.);
#16704=ORIENTED_EDGE('',*,*,#12705,.F.);
#16705=ORIENTED_EDGE('',*,*,#12893,.T.);
#16706=ORIENTED_EDGE('',*,*,#12909,.T.);
#16707=ORIENTED_EDGE('',*,*,#12704,.F.);
#16708=ORIENTED_EDGE('',*,*,#12896,.T.);
#16709=ORIENTED_EDGE('',*,*,#12894,.T.);
#16710=ORIENTED_EDGE('',*,*,#12703,.F.);
#16711=ORIENTED_EDGE('',*,*,#12899,.T.);
#16712=ORIENTED_EDGE('',*,*,#12897,.T.);
#16713=ORIENTED_EDGE('',*,*,#12708,.F.);
#16714=ORIENTED_EDGE('',*,*,#12902,.T.);
#16715=ORIENTED_EDGE('',*,*,#12900,.T.);
#16716=ORIENTED_EDGE('',*,*,#12707,.F.);
#16717=ORIENTED_EDGE('',*,*,#12905,.T.);
#16718=ORIENTED_EDGE('',*,*,#12903,.T.);
#16719=ORIENTED_EDGE('',*,*,#12706,.F.);
#16720=ORIENTED_EDGE('',*,*,#12908,.T.);
#16721=ORIENTED_EDGE('',*,*,#12906,.T.);
#16722=ORIENTED_EDGE('',*,*,#12701,.F.);
#16723=ORIENTED_EDGE('',*,*,#12696,.T.);
#16724=ORIENTED_EDGE('',*,*,#12698,.F.);
#16725=ORIENTED_EDGE('',*,*,#12693,.T.);
#16726=ORIENTED_EDGE('',*,*,#12690,.T.);
#16727=ORIENTED_EDGE('',*,*,#12695,.F.);
#16728=ORIENTED_EDGE('',*,*,#12687,.T.);
#16729=ORIENTED_EDGE('',*,*,#12692,.F.);
#22776=CYLINDRICAL_SURFACE('',#25058,4.49999999999999);
#22777=CYLINDRICAL_SURFACE('',#25061,4.49999999999999);
#22778=CYLINDRICAL_SURFACE('',#25064,12.);
#22779=CYLINDRICAL_SURFACE('',#25067,7.75);
#22780=CYLINDRICAL_SURFACE('',#25070,6.00000000000001);
#22781=CYLINDRICAL_SURFACE('',#25073,7.74999999999999);
#22782=CYLINDRICAL_SURFACE('',#25076,12.);
#22783=CYLINDRICAL_SURFACE('',#25107,3.1);
#22784=CYLINDRICAL_SURFACE('',#25110,3.1);
#22785=CYLINDRICAL_SURFACE('',#25113,3.1);
#22786=CYLINDRICAL_SURFACE('',#25116,3.1);
#22787=CYLINDRICAL_SURFACE('',#25119,3.5);
#22788=CYLINDRICAL_SURFACE('',#25122,3.5);
#22789=CYLINDRICAL_SURFACE('',#25125,3.50000000000001);
#22790=CYLINDRICAL_SURFACE('',#25128,3.50000000000001);
#23231=ADVANCED_FACE('',(#2239),#22776,.F.);
#23232=ADVANCED_FACE('',(#2240),#22777,.F.);
#23233=ADVANCED_FACE('',(#2241),#22778,.F.);
#23234=ADVANCED_FACE('',(#2242),#22779,.F.);
#23235=ADVANCED_FACE('',(#2243),#22780,.F.);
#23236=ADVANCED_FACE('',(#2244),#22781,.F.);
#23237=ADVANCED_FACE('',(#2245),#22782,.F.);
#23238=ADVANCED_FACE('',(#2246),#2114,.F.);
#23239=ADVANCED_FACE('',(#2247),#2115,.F.);
#23240=ADVANCED_FACE('',(#2248),#2116,.F.);
#23241=ADVANCED_FACE('',(#2249),#2117,.F.);
#23242=ADVANCED_FACE('',(#2250),#22783,.T.);
#23243=ADVANCED_FACE('',(#2251),#22784,.T.);
#23244=ADVANCED_FACE('',(#2252),#22785,.T.);
#23245=ADVANCED_FACE('',(#2253),#22786,.T.);
#23246=ADVANCED_FACE('',(#2254),#22787,.F.);
#23247=ADVANCED_FACE('',(#2255),#22788,.F.);
#23248=ADVANCED_FACE('',(#2256),#22789,.F.);
#23249=ADVANCED_FACE('',(#2257),#22790,.F.);
#23250=ADVANCED_FACE('',(#2258,#1046),#1371,.T.);
#23251=ADVANCED_FACE('',(#2259,#1047),#1372,.T.);
#23252=ADVANCED_FACE('',(#2260,#1048),#1373,.T.);
#23253=ADVANCED_FACE('',(#2261,#1049),#1374,.T.);
#23254=ADVANCED_FACE('',(#2262,#1050),#1375,.T.);
#23255=ADVANCED_FACE('',(#2263,#1051),#1376,.F.);
#23256=ADVANCED_FACE('',(#2264),#1377,.F.);
#23257=ADVANCED_FACE('',(#2265),#1378,.F.);
#23258=ADVANCED_FACE('',(#2266,#1052,#1053),#1379,.F.);
#23259=ADVANCED_FACE('',(#2267),#1380,.F.);
#23260=ADVANCED_FACE('',(#2268),#1381,.F.);
#23261=ADVANCED_FACE('',(#2269,#1054),#1382,.F.);
#23262=ADVANCED_FACE('',(#2270),#1383,.F.);
#23263=ADVANCED_FACE('',(#2271),#1384,.F.);
#23264=ADVANCED_FACE('',(#2272),#1385,.F.);
#23265=ADVANCED_FACE('',(#2273),#1386,.F.);
#23266=ADVANCED_FACE('',(#2274),#1387,.F.);
#23267=ADVANCED_FACE('',(#2275,#1055),#1388,.F.);
#23268=ADVANCED_FACE('',(#2276,#1056,#1057,#1058,#1059,#1060),#1389,.F.);
#23269=ADVANCED_FACE('',(#2277),#1390,.F.);
#23270=ADVANCED_FACE('',(#2278),#1391,.F.);
#23271=ADVANCED_FACE('',(#2279),#1392,.F.);
#23272=ADVANCED_FACE('',(#2280),#1393,.F.);
#23273=ADVANCED_FACE('',(#2281),#1394,.F.);
#23274=ADVANCED_FACE('',(#2282),#1395,.F.);
#23275=ADVANCED_FACE('',(#2283),#1396,.F.);
#23276=ADVANCED_FACE('',(#2284),#1397,.F.);
#23277=ADVANCED_FACE('',(#2285,#1061),#1398,.T.);
#23278=ADVANCED_FACE('',(#2286,#1062),#1399,.T.);
#23279=ADVANCED_FACE('',(#2287,#1063),#1400,.T.);
#23280=ADVANCED_FACE('',(#2288,#1064),#1401,.T.);
#23281=ADVANCED_FACE('',(#2289),#1402,.F.);
#23282=ADVANCED_FACE('',(#2290),#1403,.F.);
#23283=ADVANCED_FACE('',(#2291),#1404,.F.);
#23284=ADVANCED_FACE('',(#2292),#1405,.F.);
#23285=ADVANCED_FACE('',(#2293),#1406,.F.);
#23286=ADVANCED_FACE('',(#2294),#1407,.F.);
#23287=ADVANCED_FACE('',(#2295),#1408,.T.);
#23288=ADVANCED_FACE('',(#2296),#1409,.T.);
#23289=ADVANCED_FACE('',(#2297),#1410,.T.);
#23290=ADVANCED_FACE('',(#2298),#1411,.T.);
#23291=ADVANCED_FACE('',(#2299),#1412,.T.);
#23292=ADVANCED_FACE('',(#2300),#1413,.T.);
#23293=ADVANCED_FACE('',(#2301),#1414,.F.);
#23294=ADVANCED_FACE('',(#2302),#1415,.F.);
#23295=ADVANCED_FACE('',(#2303),#1416,.F.);
#23296=ADVANCED_FACE('',(#2304),#1417,.F.);
#23297=ADVANCED_FACE('',(#2305),#1418,.F.);
#23298=ADVANCED_FACE('',(#2306),#1419,.F.);
#23299=ADVANCED_FACE('',(#2307),#1420,.T.);
#23300=ADVANCED_FACE('',(#2308),#1421,.T.);
#23301=ADVANCED_FACE('',(#2309),#1422,.T.);
#23302=ADVANCED_FACE('',(#2310),#1423,.T.);
#23303=ADVANCED_FACE('',(#2311),#1424,.T.);
#23304=ADVANCED_FACE('',(#2312),#1425,.T.);
#23305=ADVANCED_FACE('',(#2313),#1426,.F.);
#23306=ADVANCED_FACE('',(#2314),#1427,.F.);
#23307=ADVANCED_FACE('',(#2315),#1428,.F.);
#23308=ADVANCED_FACE('',(#2316),#1429,.F.);
#23309=ADVANCED_FACE('',(#2317),#1430,.F.);
#23310=ADVANCED_FACE('',(#2318),#1431,.F.);
#23311=ADVANCED_FACE('',(#2319),#1432,.T.);
#23312=ADVANCED_FACE('',(#2320),#1433,.T.);
#23313=ADVANCED_FACE('',(#2321),#1434,.T.);
#23314=ADVANCED_FACE('',(#2322),#1435,.T.);
#23315=ADVANCED_FACE('',(#2323),#1436,.T.);
#23316=ADVANCED_FACE('',(#2324),#1437,.T.);
#23317=ADVANCED_FACE('',(#2325),#1438,.F.);
#23318=ADVANCED_FACE('',(#2326),#1439,.F.);
#23319=ADVANCED_FACE('',(#2327),#1440,.F.);
#23320=ADVANCED_FACE('',(#2328),#1441,.F.);
#23321=ADVANCED_FACE('',(#2329),#1442,.F.);
#23322=ADVANCED_FACE('',(#2330),#1443,.F.);
#23323=ADVANCED_FACE('',(#2331),#1444,.T.);
#23324=ADVANCED_FACE('',(#2332),#1445,.T.);
#23325=ADVANCED_FACE('',(#2333),#1446,.T.);
#23326=ADVANCED_FACE('',(#2334),#1447,.T.);
#23327=ADVANCED_FACE('',(#2335),#1448,.T.);
#23328=ADVANCED_FACE('',(#2336),#1449,.T.);
#23329=ADVANCED_FACE('',(#2337,#1065),#1450,.F.);
#23330=ADVANCED_FACE('',(#2338,#1066),#1451,.F.);
#23331=ADVANCED_FACE('',(#2339,#1067),#1452,.F.);
#23332=ADVANCED_FACE('',(#2340,#1068),#1453,.F.);
#24529=CLOSED_SHELL('',(#23231,#23232,#23233,#23234,#23235,#23236,#23237,
#23238,#23239,#23240,#23241,#23242,#23243,#23244,#23245,#23246,#23247,#23248,
#23249,#23250,#23251,#23252,#23253,#23254,#23255,#23256,#23257,#23258,#23259,
#23260,#23261,#23262,#23263,#23264,#23265,#23266,#23267,#23268,#23269,#23270,
#23271,#23272,#23273,#23274,#23275,#23276,#23277,#23278,#23279,#23280,#23281,
#23282,#23283,#23284,#23285,#23286,#23287,#23288,#23289,#23290,#23291,#23292,
#23293,#23294,#23295,#23296,#23297,#23298,#23299,#23300,#23301,#23302,#23303,
#23304,#23305,#23306,#23307,#23308,#23309,#23310,#23311,#23312,#23313,#23314,
#23315,#23316,#23317,#23318,#23319,#23320,#23321,#23322,#23323,#23324,#23325,
#23326,#23327,#23328,#23329,#23330,#23331,#23332));
#25057=AXIS2_PLACEMENT_3D('',#35178,#27905,#27906);
#25058=AXIS2_PLACEMENT_3D('',#35179,#27907,#27908);
#25059=AXIS2_PLACEMENT_3D('',#35181,#27909,#27910);
#25060=AXIS2_PLACEMENT_3D('',#35184,#27912,#27913);
#25061=AXIS2_PLACEMENT_3D('',#35185,#27914,#27915);
#25062=AXIS2_PLACEMENT_3D('',#35187,#27916,#27917);
#25063=AXIS2_PLACEMENT_3D('',#35190,#27919,#27920);
#25064=AXIS2_PLACEMENT_3D('',#35191,#27921,#27922);
#25065=AXIS2_PLACEMENT_3D('',#35193,#27923,#27924);
#25066=AXIS2_PLACEMENT_3D('',#35196,#27926,#27927);
#25067=AXIS2_PLACEMENT_3D('',#35197,#27928,#27929);
#25068=AXIS2_PLACEMENT_3D('',#35199,#27930,#27931);
#25069=AXIS2_PLACEMENT_3D('',#35202,#27933,#27934);
#25070=AXIS2_PLACEMENT_3D('',#35203,#27935,#27936);
#25071=AXIS2_PLACEMENT_3D('',#35205,#27937,#27938);
#25072=AXIS2_PLACEMENT_3D('',#35208,#27940,#27941);
#25073=AXIS2_PLACEMENT_3D('',#35209,#27942,#27943);
#25074=AXIS2_PLACEMENT_3D('',#35211,#27944,#27945);
#25075=AXIS2_PLACEMENT_3D('',#35214,#27947,#27948);
#25076=AXIS2_PLACEMENT_3D('',#35215,#27949,#27950);
#25077=AXIS2_PLACEMENT_3D('',#35217,#27951,#27952);
#25078=AXIS2_PLACEMENT_3D('',#35220,#27954,#27955);
#25079=AXIS2_PLACEMENT_3D('',#35221,#27956,#27957);
#25080=AXIS2_PLACEMENT_3D('',#35226,#27959,#27960);
#25081=AXIS2_PLACEMENT_3D('',#35228,#27961,#27962);
#25082=AXIS2_PLACEMENT_3D('',#35230,#27963,#27964);
#25083=AXIS2_PLACEMENT_3D('',#35232,#27965,#27966);
#25084=AXIS2_PLACEMENT_3D('',#35234,#27967,#27968);
#25085=AXIS2_PLACEMENT_3D('',#35235,#27969,#27970);
#25086=AXIS2_PLACEMENT_3D('',#35236,#27971,#27972);
#25087=AXIS2_PLACEMENT_3D('',#35241,#27974,#27975);
#25088=AXIS2_PLACEMENT_3D('',#35243,#27976,#27977);
#25089=AXIS2_PLACEMENT_3D('',#35245,#27978,#27979);
#25090=AXIS2_PLACEMENT_3D('',#35247,#27980,#27981);
#25091=AXIS2_PLACEMENT_3D('',#35249,#27982,#27983);
#25092=AXIS2_PLACEMENT_3D('',#35250,#27984,#27985);
#25093=AXIS2_PLACEMENT_3D('',#35251,#27986,#27987);
#25094=AXIS2_PLACEMENT_3D('',#35256,#27989,#27990);
#25095=AXIS2_PLACEMENT_3D('',#35258,#27991,#27992);
#25096=AXIS2_PLACEMENT_3D('',#35260,#27993,#27994);
#25097=AXIS2_PLACEMENT_3D('',#35262,#27995,#27996);
#25098=AXIS2_PLACEMENT_3D('',#35264,#27997,#27998);
#25099=AXIS2_PLACEMENT_3D('',#35265,#27999,#28000);
#25100=AXIS2_PLACEMENT_3D('',#35266,#28001,#28002);
#25101=AXIS2_PLACEMENT_3D('',#35271,#28004,#28005);
#25102=AXIS2_PLACEMENT_3D('',#35273,#28006,#28007);
#25103=AXIS2_PLACEMENT_3D('',#35275,#28008,#28009);
#25104=AXIS2_PLACEMENT_3D('',#35277,#28010,#28011);
#25105=AXIS2_PLACEMENT_3D('',#35279,#28012,#28013);
#25106=AXIS2_PLACEMENT_3D('',#35280,#28014,#28015);
#25107=AXIS2_PLACEMENT_3D('',#35281,#28016,#28017);
#25108=AXIS2_PLACEMENT_3D('',#35283,#28018,#28019);
#25109=AXIS2_PLACEMENT_3D('',#35286,#28021,#28022);
#25110=AXIS2_PLACEMENT_3D('',#35287,#28023,#28024);
#25111=AXIS2_PLACEMENT_3D('',#35289,#28025,#28026);
#25112=AXIS2_PLACEMENT_3D('',#35292,#28028,#28029);
#25113=AXIS2_PLACEMENT_3D('',#35293,#28030,#28031);
#25114=AXIS2_PLACEMENT_3D('',#35295,#28032,#28033);
#25115=AXIS2_PLACEMENT_3D('',#35298,#28035,#28036);
#25116=AXIS2_PLACEMENT_3D('',#35299,#28037,#28038);
#25117=AXIS2_PLACEMENT_3D('',#35301,#28039,#28040);
#25118=AXIS2_PLACEMENT_3D('',#35304,#28042,#28043);
#25119=AXIS2_PLACEMENT_3D('',#35305,#28044,#28045);
#25120=AXIS2_PLACEMENT_3D('',#35307,#28046,#28047);
#25121=AXIS2_PLACEMENT_3D('',#35310,#28049,#28050);
#25122=AXIS2_PLACEMENT_3D('',#35311,#28051,#28052);
#25123=AXIS2_PLACEMENT_3D('',#35313,#28053,#28054);
#25124=AXIS2_PLACEMENT_3D('',#35316,#28056,#28057);
#25125=AXIS2_PLACEMENT_3D('',#35317,#28058,#28059);
#25126=AXIS2_PLACEMENT_3D('',#35319,#28060,#28061);
#25127=AXIS2_PLACEMENT_3D('',#35322,#28063,#28064);
#25128=AXIS2_PLACEMENT_3D('',#35323,#28065,#28066);
#25129=AXIS2_PLACEMENT_3D('',#35325,#28067,#28068);
#25130=AXIS2_PLACEMENT_3D('',#35328,#28070,#28071);
#25131=AXIS2_PLACEMENT_3D('',#35329,#28072,#28073);
#25132=AXIS2_PLACEMENT_3D('',#35330,#28074,#28075);
#25133=AXIS2_PLACEMENT_3D('',#35331,#28076,#28077);
#25134=AXIS2_PLACEMENT_3D('',#35332,#28078,#28079);
#25135=AXIS2_PLACEMENT_3D('',#35333,#28080,#28081);
#25136=AXIS2_PLACEMENT_3D('',#35374,#28102,#28103);
#25137=AXIS2_PLACEMENT_3D('',#35380,#28107,#28108);
#25138=AXIS2_PLACEMENT_3D('',#35384,#28111,#28112);
#25139=AXIS2_PLACEMENT_3D('',#35388,#28115,#28116);
#25140=AXIS2_PLACEMENT_3D('',#35392,#28119,#28120);
#25141=AXIS2_PLACEMENT_3D('',#35396,#28123,#28124);
#25142=AXIS2_PLACEMENT_3D('',#35400,#28127,#28128);
#25143=AXIS2_PLACEMENT_3D('',#35404,#28131,#28132);
#25144=AXIS2_PLACEMENT_3D('',#35408,#28135,#28136);
#25145=AXIS2_PLACEMENT_3D('',#35412,#28139,#28140);
#25146=AXIS2_PLACEMENT_3D('',#35416,#28143,#28144);
#25147=AXIS2_PLACEMENT_3D('',#35420,#28147,#28148);
#25148=AXIS2_PLACEMENT_3D('',#35422,#28150,#28151);
#25149=AXIS2_PLACEMENT_3D('',#35423,#28152,#28153);
#25150=AXIS2_PLACEMENT_3D('',#35440,#28162,#28163);
#25151=AXIS2_PLACEMENT_3D('',#35443,#28166,#28167);
#25152=AXIS2_PLACEMENT_3D('',#35445,#28169,#28170);
#25153=AXIS2_PLACEMENT_3D('',#35447,#28172,#28173);
#25154=AXIS2_PLACEMENT_3D('',#35449,#28175,#28176);
#25155=AXIS2_PLACEMENT_3D('',#35451,#28178,#28179);
#25156=AXIS2_PLACEMENT_3D('',#35453,#28181,#28182);
#25157=AXIS2_PLACEMENT_3D('',#35455,#28184,#28185);
#25158=AXIS2_PLACEMENT_3D('',#35456,#28186,#28187);
#25159=AXIS2_PLACEMENT_3D('',#35469,#28194,#28195);
#25160=AXIS2_PLACEMENT_3D('',#35482,#28202,#28203);
#25161=AXIS2_PLACEMENT_3D('',#35495,#28210,#28211);
#25162=AXIS2_PLACEMENT_3D('',#35508,#28218,#28219);
#25163=AXIS2_PLACEMENT_3D('',#35515,#28224,#28225);
#25164=AXIS2_PLACEMENT_3D('',#35520,#28229,#28230);
#25165=AXIS2_PLACEMENT_3D('',#35525,#28234,#28235);
#25166=AXIS2_PLACEMENT_3D('',#35530,#28239,#28240);
#25167=AXIS2_PLACEMENT_3D('',#35535,#28244,#28245);
#25168=AXIS2_PLACEMENT_3D('',#35538,#28248,#28249);
#25169=AXIS2_PLACEMENT_3D('',#35539,#28250,#28251);
#25170=AXIS2_PLACEMENT_3D('',#35540,#28252,#28253);
#25171=AXIS2_PLACEMENT_3D('',#35541,#28254,#28255);
#25172=AXIS2_PLACEMENT_3D('',#35542,#28256,#28257);
#25173=AXIS2_PLACEMENT_3D('',#35543,#28258,#28259);
#25174=AXIS2_PLACEMENT_3D('',#35544,#28260,#28261);
#25175=AXIS2_PLACEMENT_3D('',#35551,#28266,#28267);
#25176=AXIS2_PLACEMENT_3D('',#35556,#28271,#28272);
#25177=AXIS2_PLACEMENT_3D('',#35561,#28276,#28277);
#25178=AXIS2_PLACEMENT_3D('',#35566,#28281,#28282);
#25179=AXIS2_PLACEMENT_3D('',#35571,#28286,#28287);
#25180=AXIS2_PLACEMENT_3D('',#35574,#28290,#28291);
#25181=AXIS2_PLACEMENT_3D('',#35575,#28292,#28293);
#25182=AXIS2_PLACEMENT_3D('',#35576,#28294,#28295);
#25183=AXIS2_PLACEMENT_3D('',#35577,#28296,#28297);
#25184=AXIS2_PLACEMENT_3D('',#35578,#28298,#28299);
#25185=AXIS2_PLACEMENT_3D('',#35579,#28300,#28301);
#25186=AXIS2_PLACEMENT_3D('',#35580,#28302,#28303);
#25187=AXIS2_PLACEMENT_3D('',#35587,#28308,#28309);
#25188=AXIS2_PLACEMENT_3D('',#35592,#28313,#28314);
#25189=AXIS2_PLACEMENT_3D('',#35597,#28318,#28319);
#25190=AXIS2_PLACEMENT_3D('',#35602,#28323,#28324);
#25191=AXIS2_PLACEMENT_3D('',#35607,#28328,#28329);
#25192=AXIS2_PLACEMENT_3D('',#35610,#28332,#28333);
#25193=AXIS2_PLACEMENT_3D('',#35611,#28334,#28335);
#25194=AXIS2_PLACEMENT_3D('',#35612,#28336,#28337);
#25195=AXIS2_PLACEMENT_3D('',#35613,#28338,#28339);
#25196=AXIS2_PLACEMENT_3D('',#35614,#28340,#28341);
#25197=AXIS2_PLACEMENT_3D('',#35615,#28342,#28343);
#25198=AXIS2_PLACEMENT_3D('',#35616,#28344,#28345);
#25199=AXIS2_PLACEMENT_3D('',#35623,#28350,#28351);
#25200=AXIS2_PLACEMENT_3D('',#35628,#28355,#28356);
#25201=AXIS2_PLACEMENT_3D('',#35633,#28360,#28361);
#25202=AXIS2_PLACEMENT_3D('',#35638,#28365,#28366);
#25203=AXIS2_PLACEMENT_3D('',#35643,#28370,#28371);
#25204=AXIS2_PLACEMENT_3D('',#35646,#28374,#28375);
#25205=AXIS2_PLACEMENT_3D('',#35647,#28376,#28377);
#25206=AXIS2_PLACEMENT_3D('',#35648,#28378,#28379);
#25207=AXIS2_PLACEMENT_3D('',#35649,#28380,#28381);
#25208=AXIS2_PLACEMENT_3D('',#35650,#28382,#28383);
#25209=AXIS2_PLACEMENT_3D('',#35651,#28384,#28385);
#25210=AXIS2_PLACEMENT_3D('',#35652,#28386,#28387);
#25211=AXIS2_PLACEMENT_3D('',#35653,#28388,#28389);
#25212=AXIS2_PLACEMENT_3D('',#35654,#28390,#28391);
#25213=AXIS2_PLACEMENT_3D('',#35655,#28392,#28393);
#27905=DIRECTION('axis',(0.,0.,1.));
#27906=DIRECTION('refdir',(1.,0.,0.));
#27907=DIRECTION('center_axis',(0.,1.,3.01691039300315E-16));
#27908=DIRECTION('ref_axis',(0.,-3.01691039300315E-16,1.));
#27909=DIRECTION('center_axis',(0.,1.,3.01691039300315E-16));
#27910=DIRECTION('ref_axis',(0.,-3.01691039300315E-16,1.));
#27911=DIRECTION('',(0.,1.,3.01691039300315E-16));
#27912=DIRECTION('center_axis',(0.,1.,3.01691039300315E-16));
#27913=DIRECTION('ref_axis',(0.,-3.01691039300315E-16,1.));
#27914=DIRECTION('center_axis',(0.,1.,3.01691039300315E-16));
#27915=DIRECTION('ref_axis',(0.,-3.01691039300315E-16,1.));
#27916=DIRECTION('center_axis',(0.,1.,3.01691039300315E-16));
#27917=DIRECTION('ref_axis',(0.,-3.01691039300315E-16,1.));
#27918=DIRECTION('',(0.,1.,3.01691039300315E-16));
#27919=DIRECTION('center_axis',(0.,1.,3.01691039300315E-16));
#27920=DIRECTION('ref_axis',(0.,-3.01691039300315E-16,1.));
#27921=DIRECTION('center_axis',(1.,0.,0.));
#27922=DIRECTION('ref_axis',(0.,0.,-1.));
#27923=DIRECTION('center_axis',(1.,0.,0.));
#27924=DIRECTION('ref_axis',(0.,0.,-1.));
#27925=DIRECTION('',(1.,0.,0.));
#27926=DIRECTION('center_axis',(1.,0.,0.));
#27927=DIRECTION('ref_axis',(0.,0.,-1.));
#27928=DIRECTION('center_axis',(1.,0.,0.));
#27929=DIRECTION('ref_axis',(0.,0.,-1.));
#27930=DIRECTION('center_axis',(1.,0.,0.));
#27931=DIRECTION('ref_axis',(0.,0.,-1.));
#27932=DIRECTION('',(1.,0.,0.));
#27933=DIRECTION('center_axis',(1.,0.,0.));
#27934=DIRECTION('ref_axis',(0.,0.,-1.));
#27935=DIRECTION('center_axis',(1.,0.,0.));
#27936=DIRECTION('ref_axis',(0.,0.,-1.));
#27937=DIRECTION('center_axis',(1.,0.,0.));
#27938=DIRECTION('ref_axis',(0.,0.,-1.));
#27939=DIRECTION('',(1.,0.,0.));
#27940=DIRECTION('center_axis',(1.,0.,0.));
#27941=DIRECTION('ref_axis',(0.,0.,-1.));
#27942=DIRECTION('center_axis',(1.,0.,0.));
#27943=DIRECTION('ref_axis',(0.,0.,-1.));
#27944=DIRECTION('center_axis',(1.,0.,0.));
#27945=DIRECTION('ref_axis',(0.,0.,-1.));
#27946=DIRECTION('',(1.,0.,0.));
#27947=DIRECTION('center_axis',(1.,0.,0.));
#27948=DIRECTION('ref_axis',(0.,0.,-1.));
#27949=DIRECTION('center_axis',(1.,0.,0.));
#27950=DIRECTION('ref_axis',(0.,0.,-1.));
#27951=DIRECTION('center_axis',(1.,0.,0.));
#27952=DIRECTION('ref_axis',(0.,0.,-1.));
#27953=DIRECTION('',(1.,0.,0.));
#27954=DIRECTION('center_axis',(1.,0.,0.));
#27955=DIRECTION('ref_axis',(0.,0.,-1.));
#27956=DIRECTION('center_axis',(1.,0.,0.));
#27957=DIRECTION('ref_axis',(0.,0.,-1.));
#27958=DIRECTION('',(0.515038074910055,-1.04972719113862E-16,0.857167300702111));
#27959=DIRECTION('center_axis',(1.,0.,0.));
#27960=DIRECTION('ref_axis',(0.,0.,-1.));
#27961=DIRECTION('center_axis',(1.,0.,0.));
#27962=DIRECTION('ref_axis',(0.,0.,-1.));
#27963=DIRECTION('center_axis',(1.,0.,0.));
#27964=DIRECTION('ref_axis',(0.,0.,-1.));
#27965=DIRECTION('center_axis',(1.,0.,0.));
#27966=DIRECTION('ref_axis',(0.,0.,-1.));
#27967=DIRECTION('center_axis',(1.,0.,0.));
#27968=DIRECTION('ref_axis',(0.,0.,-1.));
#27969=DIRECTION('center_axis',(1.,0.,0.));
#27970=DIRECTION('ref_axis',(0.,0.,-1.));
#27971=DIRECTION('center_axis',(1.,0.,0.));
#27972=DIRECTION('ref_axis',(0.,0.,-1.));
#27973=DIRECTION('',(0.515038074910055,-1.04972719113862E-16,0.857167300702111));
#27974=DIRECTION('center_axis',(1.,0.,0.));
#27975=DIRECTION('ref_axis',(0.,0.,-1.));
#27976=DIRECTION('center_axis',(1.,0.,0.));
#27977=DIRECTION('ref_axis',(0.,0.,-1.));
#27978=DIRECTION('center_axis',(1.,0.,0.));
#27979=DIRECTION('ref_axis',(0.,0.,-1.));
#27980=DIRECTION('center_axis',(1.,0.,0.));
#27981=DIRECTION('ref_axis',(0.,0.,-1.));
#27982=DIRECTION('center_axis',(1.,0.,0.));
#27983=DIRECTION('ref_axis',(0.,0.,-1.));
#27984=DIRECTION('center_axis',(1.,0.,0.));
#27985=DIRECTION('ref_axis',(0.,0.,-1.));
#27986=DIRECTION('center_axis',(1.,0.,0.));
#27987=DIRECTION('ref_axis',(0.,0.,-1.));
#27988=DIRECTION('',(0.515038074910055,-1.04972719113862E-16,0.857167300702112));
#27989=DIRECTION('center_axis',(1.,0.,0.));
#27990=DIRECTION('ref_axis',(0.,0.,-1.));
#27991=DIRECTION('center_axis',(1.,0.,0.));
#27992=DIRECTION('ref_axis',(0.,0.,-1.));
#27993=DIRECTION('center_axis',(1.,0.,0.));
#27994=DIRECTION('ref_axis',(0.,0.,-1.));
#27995=DIRECTION('center_axis',(1.,0.,0.));
#27996=DIRECTION('ref_axis',(0.,0.,-1.));
#27997=DIRECTION('center_axis',(1.,0.,0.));
#27998=DIRECTION('ref_axis',(0.,0.,-1.));
#27999=DIRECTION('center_axis',(1.,0.,0.));
#28000=DIRECTION('ref_axis',(0.,0.,-1.));
#28001=DIRECTION('center_axis',(1.,0.,0.));
#28002=DIRECTION('ref_axis',(0.,0.,-1.));
#28003=DIRECTION('',(0.515038074910055,-1.04972719113862E-16,0.857167300702112));
#28004=DIRECTION('center_axis',(1.,0.,0.));
#28005=DIRECTION('ref_axis',(0.,0.,-1.));
#28006=DIRECTION('center_axis',(1.,0.,0.));
#28007=DIRECTION('ref_axis',(0.,0.,-1.));
#28008=DIRECTION('center_axis',(1.,0.,0.));
#28009=DIRECTION('ref_axis',(0.,0.,-1.));
#28010=DIRECTION('center_axis',(1.,0.,0.));
#28011=DIRECTION('ref_axis',(0.,0.,-1.));
#28012=DIRECTION('center_axis',(1.,0.,0.));
#28013=DIRECTION('ref_axis',(0.,0.,-1.));
#28014=DIRECTION('center_axis',(1.,0.,0.));
#28015=DIRECTION('ref_axis',(0.,0.,-1.));
#28016=DIRECTION('center_axis',(-1.,0.,0.));
#28017=DIRECTION('ref_axis',(0.,0.,1.));
#28018=DIRECTION('center_axis',(1.,0.,0.));
#28019=DIRECTION('ref_axis',(0.,0.,-1.));
#28020=DIRECTION('',(1.,0.,0.));
#28021=DIRECTION('center_axis',(1.,0.,0.));
#28022=DIRECTION('ref_axis',(0.,0.,-1.));
#28023=DIRECTION('center_axis',(-1.,0.,0.));
#28024=DIRECTION('ref_axis',(0.,0.,1.));
#28025=DIRECTION('center_axis',(1.,0.,0.));
#28026=DIRECTION('ref_axis',(0.,0.,-1.));
#28027=DIRECTION('',(1.,0.,0.));
#28028=DIRECTION('center_axis',(1.,0.,0.));
#28029=DIRECTION('ref_axis',(0.,0.,-1.));
#28030=DIRECTION('center_axis',(-1.,0.,0.));
#28031=DIRECTION('ref_axis',(0.,0.,1.));
#28032=DIRECTION('center_axis',(1.,0.,0.));
#28033=DIRECTION('ref_axis',(0.,0.,-1.));
#28034=DIRECTION('',(1.,0.,0.));
#28035=DIRECTION('center_axis',(1.,0.,0.));
#28036=DIRECTION('ref_axis',(0.,0.,-1.));
#28037=DIRECTION('center_axis',(-1.,0.,0.));
#28038=DIRECTION('ref_axis',(0.,0.,1.));
#28039=DIRECTION('center_axis',(1.,0.,0.));
#28040=DIRECTION('ref_axis',(0.,0.,-1.));
#28041=DIRECTION('',(1.,0.,0.));
#28042=DIRECTION('center_axis',(1.,0.,0.));
#28043=DIRECTION('ref_axis',(0.,0.,-1.));
#28044=DIRECTION('center_axis',(-1.,0.,0.));
#28045=DIRECTION('ref_axis',(0.,0.,1.));
#28046=DIRECTION('center_axis',(1.,0.,0.));
#28047=DIRECTION('ref_axis',(0.,0.,-1.));
#28048=DIRECTION('',(-1.,0.,0.));
#28049=DIRECTION('center_axis',(-1.,0.,0.));
#28050=DIRECTION('ref_axis',(0.,0.,-1.));
#28051=DIRECTION('center_axis',(-1.,0.,0.));
#28052=DIRECTION('ref_axis',(0.,0.,1.));
#28053=DIRECTION('center_axis',(1.,0.,0.));
#28054=DIRECTION('ref_axis',(0.,0.,-1.));
#28055=DIRECTION('',(-1.,0.,0.));
#28056=DIRECTION('center_axis',(-1.,0.,0.));
#28057=DIRECTION('ref_axis',(0.,0.,-1.));
#28058=DIRECTION('center_axis',(-1.,0.,0.));
#28059=DIRECTION('ref_axis',(0.,0.,1.));
#28060=DIRECTION('center_axis',(1.,0.,0.));
#28061=DIRECTION('ref_axis',(0.,0.,-1.));
#28062=DIRECTION('',(-1.,0.,0.));
#28063=DIRECTION('center_axis',(-1.,0.,0.));
#28064=DIRECTION('ref_axis',(0.,0.,-1.));
#28065=DIRECTION('center_axis',(-1.,0.,0.));
#28066=DIRECTION('ref_axis',(0.,0.,1.));
#28067=DIRECTION('center_axis',(1.,0.,0.));
#28068=DIRECTION('ref_axis',(0.,0.,-1.));
#28069=DIRECTION('',(-1.,0.,0.));
#28070=DIRECTION('center_axis',(-1.,0.,0.));
#28071=DIRECTION('ref_axis',(0.,0.,-1.));
#28072=DIRECTION('center_axis',(1.,0.,0.));
#28073=DIRECTION('ref_axis',(0.,0.,-1.));
#28074=DIRECTION('center_axis',(1.,0.,0.));
#28075=DIRECTION('ref_axis',(0.,0.,-1.));
#28076=DIRECTION('center_axis',(1.,0.,0.));
#28077=DIRECTION('ref_axis',(0.,0.,-1.));
#28078=DIRECTION('center_axis',(1.,0.,0.));
#28079=DIRECTION('ref_axis',(0.,0.,-1.));
#28080=DIRECTION('center_axis',(1.,0.,0.));
#28081=DIRECTION('ref_axis',(0.,0.,-1.));
#28082=DIRECTION('',(0.,-2.10269512239613E-16,1.));
#28083=DIRECTION('',(0.,-0.707106781186582,0.707106781186513));
#28084=DIRECTION('',(0.,-1.,-2.95272081017329E-16));
#28085=DIRECTION('',(0.,2.55331806268467E-16,-1.));
#28086=DIRECTION('',(0.,1.,5.90544162034659E-16));
#28087=DIRECTION('',(0.,0.707106781186562,0.707106781186533));
#28088=DIRECTION('',(0.,2.10269512239613E-16,1.));
#28089=DIRECTION('',(0.,1.,1.87537673078574E-16));
#28090=DIRECTION('',(0.,0.70710678118655,0.707106781186545));
#28091=DIRECTION('',(0.,0.,1.));
#28092=DIRECTION('',(0.,-0.707106781186543,0.707106781186552));
#28093=DIRECTION('',(0.,-1.,-7.50150692314296E-16));
#28094=DIRECTION('',(0.,-0.707106781186548,0.707106781186547));
#28095=DIRECTION('',(0.,0.,1.));
#28096=DIRECTION('',(0.,0.707106781186546,0.707106781186549));
#28097=DIRECTION('',(0.,1.,0.));
#28098=DIRECTION('',(0.,0.707106781186549,-0.707106781186546));
#28099=DIRECTION('',(0.,0.,-1.));
#28100=DIRECTION('',(0.,-0.707106781186546,-0.707106781186549));
#28101=DIRECTION('',(0.,-1.,0.));
#28102=DIRECTION('center_axis',(0.,-1.,-2.10269512239613E-16));
#28103=DIRECTION('ref_axis',(0.,2.10269512239613E-16,-1.));
#28104=DIRECTION('',(0.,-2.10269512239613E-16,1.));
#28105=DIRECTION('',(-1.,0.,0.));
#28106=DIRECTION('',(-1.,0.,0.));
#28107=DIRECTION('center_axis',(0.,-0.707106781186513,-0.707106781186582));
#28108=DIRECTION('ref_axis',(0.,0.707106781186582,-0.707106781186513));
#28109=DIRECTION('',(0.,-0.707106781186582,0.707106781186513));
#28110=DIRECTION('',(-1.,0.,0.));
#28111=DIRECTION('center_axis',(0.,2.95272081017329E-16,-1.));
#28112=DIRECTION('ref_axis',(0.,1.,2.95272081017329E-16));
#28113=DIRECTION('',(0.,-1.,-2.95272081017329E-16));
#28114=DIRECTION('',(-1.,0.,0.));
#28115=DIRECTION('center_axis',(0.,1.,2.55331806268467E-16));
#28116=DIRECTION('ref_axis',(0.,-2.55331806268467E-16,1.));
#28117=DIRECTION('',(0.,2.55331806268467E-16,-1.));
#28118=DIRECTION('',(-1.,0.,0.));
#28119=DIRECTION('center_axis',(0.,-5.90544162034659E-16,1.));
#28120=DIRECTION('ref_axis',(0.,-1.,-5.90544162034659E-16));
#28121=DIRECTION('',(0.,1.,5.90544162034659E-16));
#28122=DIRECTION('',(-1.,0.,0.));
#28123=DIRECTION('center_axis',(0.,-0.707106781186533,0.707106781186562));
#28124=DIRECTION('ref_axis',(0.,-0.707106781186562,-0.707106781186533));
#28125=DIRECTION('',(0.,0.707106781186562,0.707106781186533));
#28126=DIRECTION('',(-1.,0.,0.));
#28127=DIRECTION('center_axis',(0.,-1.,2.10269512239613E-16));
#28128=DIRECTION('ref_axis',(0.,-2.10269512239613E-16,-1.));
#28129=DIRECTION('',(0.,2.10269512239613E-16,1.));
#28130=DIRECTION('',(-1.,0.,0.));
#28131=DIRECTION('center_axis',(0.,-1.87537673078574E-16,1.));
#28132=DIRECTION('ref_axis',(0.,-1.,-1.87537673078574E-16));
#28133=DIRECTION('',(0.,1.,1.87537673078574E-16));
#28134=DIRECTION('',(-1.,0.,0.));
#28135=DIRECTION('center_axis',(0.,-0.707106781186545,0.70710678118655));
#28136=DIRECTION('ref_axis',(0.,-0.70710678118655,-0.707106781186545));
#28137=DIRECTION('',(0.,0.70710678118655,0.707106781186545));
#28138=DIRECTION('',(-1.,0.,0.));
#28139=DIRECTION('center_axis',(0.,-1.,0.));
#28140=DIRECTION('ref_axis',(0.,0.,-1.));
#28141=DIRECTION('',(0.,0.,1.));
#28142=DIRECTION('',(-1.,0.,0.));
#28143=DIRECTION('center_axis',(0.,-0.707106781186552,-0.707106781186543));
#28144=DIRECTION('ref_axis',(0.,0.707106781186543,-0.707106781186553));
#28145=DIRECTION('',(0.,-0.707106781186543,0.707106781186552));
#28146=DIRECTION('',(-1.,0.,0.));
#28147=DIRECTION('center_axis',(0.,7.50150692314296E-16,-1.));
#28148=DIRECTION('ref_axis',(0.,1.,7.50150692314296E-16));
#28149=DIRECTION('',(0.,-1.,-7.50150692314296E-16));
#28150=DIRECTION('center_axis',(1.,0.,0.));
#28151=DIRECTION('ref_axis',(0.,0.,-1.));
#28152=DIRECTION('center_axis',(-1.,0.,0.));
#28153=DIRECTION('ref_axis',(0.,0.,1.));
#28154=DIRECTION('',(0.,0.,1.));
#28155=DIRECTION('',(0.,-0.707106781186548,0.707106781186547));
#28156=DIRECTION('',(0.,-1.,0.));
#28157=DIRECTION('',(0.,-0.707106781186546,-0.707106781186549));
#28158=DIRECTION('',(0.,0.,-1.));
#28159=DIRECTION('',(0.,0.707106781186549,-0.707106781186546));
#28160=DIRECTION('',(0.,1.,0.));
#28161=DIRECTION('',(0.,0.707106781186546,0.707106781186549));
#28162=DIRECTION('center_axis',(0.,-1.,0.));
#28163=DIRECTION('ref_axis',(0.,0.,-1.));
#28164=DIRECTION('',(-1.,0.,0.));
#28165=DIRECTION('',(-1.,0.,0.));
#28166=DIRECTION('center_axis',(0.,-0.707106781186547,-0.707106781186548));
#28167=DIRECTION('ref_axis',(0.,0.707106781186548,-0.707106781186547));
#28168=DIRECTION('',(-1.,0.,0.));
#28169=DIRECTION('center_axis',(0.,0.,-1.));
#28170=DIRECTION('ref_axis',(-1.,0.,0.));
#28171=DIRECTION('',(-1.,0.,0.));
#28172=DIRECTION('center_axis',(0.,0.707106781186549,-0.707106781186546));
#28173=DIRECTION('ref_axis',(0.,0.707106781186546,0.707106781186549));
#28174=DIRECTION('',(-1.,0.,0.));
#28175=DIRECTION('center_axis',(0.,1.,0.));
#28176=DIRECTION('ref_axis',(0.,0.,1.));
#28177=DIRECTION('',(-1.,0.,0.));
#28178=DIRECTION('center_axis',(0.,0.707106781186546,0.707106781186549));
#28179=DIRECTION('ref_axis',(0.,-0.707106781186549,0.707106781186546));
#28180=DIRECTION('',(-1.,0.,0.));
#28181=DIRECTION('center_axis',(0.,0.,1.));
#28182=DIRECTION('ref_axis',(1.,0.,0.));
#28183=DIRECTION('',(-1.,0.,0.));
#28184=DIRECTION('center_axis',(0.,-0.707106781186549,0.707106781186546));
#28185=DIRECTION('ref_axis',(0.,-0.707106781186546,-0.707106781186549));
#28186=DIRECTION('center_axis',(1.,0.,0.));
#28187=DIRECTION('ref_axis',(0.,0.,-1.));
#28188=DIRECTION('',(0.,-0.499999999999999,0.866025403784439));
#28189=DIRECTION('',(0.,0.5,0.866025403784439));
#28190=DIRECTION('',(0.,1.,0.));
#28191=DIRECTION('',(0.,0.499999999999999,-0.866025403784439));
#28192=DIRECTION('',(0.,-0.5,-0.866025403784438));
#28193=DIRECTION('',(0.,-1.,0.));
#28194=DIRECTION('center_axis',(1.,0.,0.));
#28195=DIRECTION('ref_axis',(0.,0.,-1.));
#28196=DIRECTION('',(0.,-1.,-3.00462919747432E-15));
#28197=DIRECTION('',(0.,-0.500000000000008,0.866025403784434));
#28198=DIRECTION('',(0.,0.499999999999998,0.86602540378444));
#28199=DIRECTION('',(0.,1.,3.00462919747432E-15));
#28200=DIRECTION('',(0.,0.500000000000002,-0.866025403784437));
#28201=DIRECTION('',(0.,-0.499999999999997,-0.866025403784441));
#28202=DIRECTION('center_axis',(1.,0.,0.));
#28203=DIRECTION('ref_axis',(0.,0.,-1.));
#28204=DIRECTION('',(0.,-1.,1.00154306582477E-15));
#28205=DIRECTION('',(0.,-0.499999999999999,0.866025403784439));
#28206=DIRECTION('',(0.,0.5,0.866025403784438));
#28207=DIRECTION('',(0.,1.,-1.00154306582477E-15));
#28208=DIRECTION('',(0.,0.5,-0.866025403784439));
#28209=DIRECTION('',(0.,-0.500000000000002,-0.866025403784438));
#28210=DIRECTION('center_axis',(1.,0.,0.));
#28211=DIRECTION('ref_axis',(0.,0.,-1.));
#28212=DIRECTION('',(0.,-1.,1.00154306582478E-15));
#28213=DIRECTION('',(0.,-0.499999999999999,0.866025403784439));
#28214=DIRECTION('',(0.,0.500000000000002,0.866025403784438));
#28215=DIRECTION('',(0.,1.,-1.00154306582478E-15));
#28216=DIRECTION('',(0.,0.499999999999999,-0.866025403784439));
#28217=DIRECTION('',(0.,-0.500000000000002,-0.866025403784438));
#28218=DIRECTION('center_axis',(0.,-0.866025403784438,0.5));
#28219=DIRECTION('ref_axis',(0.,-0.5,-0.866025403784438));
#28220=DIRECTION('',(1.,0.,0.));
#28221=DIRECTION('',(0.,-0.5,-0.866025403784438));
#28222=DIRECTION('',(0.,-0.5,-0.866025403784438));
#28223=DIRECTION('',(1.,0.,0.));
#28224=DIRECTION('center_axis',(0.,0.,1.));
#28225=DIRECTION('ref_axis',(1.,0.,0.));
#28226=DIRECTION('',(0.,-1.,0.));
#28227=DIRECTION('',(0.,-1.,0.));
#28228=DIRECTION('',(1.,0.,0.));
#28229=DIRECTION('center_axis',(0.,0.866025403784439,0.499999999999999));
#28230=DIRECTION('ref_axis',(0.,-0.499999999999999,0.866025403784439));
#28231=DIRECTION('',(0.,-0.499999999999999,0.866025403784439));
#28232=DIRECTION('',(0.,-0.499999999999999,0.866025403784439));
#28233=DIRECTION('',(1.,0.,0.));
#28234=DIRECTION('center_axis',(0.,0.866025403784439,-0.5));
#28235=DIRECTION('ref_axis',(0.,0.5,0.866025403784439));
#28236=DIRECTION('',(0.,0.5,0.866025403784439));
#28237=DIRECTION('',(0.,0.5,0.866025403784439));
#28238=DIRECTION('',(1.,0.,0.));
#28239=DIRECTION('center_axis',(0.,0.,-1.));
#28240=DIRECTION('ref_axis',(-1.,0.,0.));
#28241=DIRECTION('',(0.,1.,0.));
#28242=DIRECTION('',(0.,1.,0.));
#28243=DIRECTION('',(1.,0.,0.));
#28244=DIRECTION('center_axis',(0.,-0.866025403784439,-0.499999999999999));
#28245=DIRECTION('ref_axis',(0.,0.499999999999999,-0.866025403784439));
#28246=DIRECTION('',(0.,0.499999999999999,-0.866025403784439));
#28247=DIRECTION('',(0.,0.499999999999999,-0.866025403784439));
#28248=DIRECTION('center_axis',(1.,0.,0.));
#28249=DIRECTION('ref_axis',(0.,0.,-1.));
#28250=DIRECTION('center_axis',(1.,0.,0.));
#28251=DIRECTION('ref_axis',(0.,0.,-1.));
#28252=DIRECTION('center_axis',(1.,0.,0.));
#28253=DIRECTION('ref_axis',(0.,0.,-1.));
#28254=DIRECTION('center_axis',(1.,0.,0.));
#28255=DIRECTION('ref_axis',(0.,0.,-1.));
#28256=DIRECTION('center_axis',(1.,0.,0.));
#28257=DIRECTION('ref_axis',(0.,0.,-1.));
#28258=DIRECTION('center_axis',(1.,0.,0.));
#28259=DIRECTION('ref_axis',(0.,0.,-1.));
#28260=DIRECTION('center_axis',(0.,-0.866025403784437,-0.500000000000002));
#28261=DIRECTION('ref_axis',(0.,0.500000000000002,-0.866025403784437));
#28262=DIRECTION('',(1.,0.,0.));
#28263=DIRECTION('',(0.,0.500000000000002,-0.866025403784437));
#28264=DIRECTION('',(0.,0.500000000000002,-0.866025403784437));
#28265=DIRECTION('',(1.,0.,0.));
#28266=DIRECTION('center_axis',(0.,-0.866025403784441,0.499999999999997));
#28267=DIRECTION('ref_axis',(0.,-0.499999999999997,-0.866025403784441));
#28268=DIRECTION('',(0.,-0.499999999999997,-0.866025403784441));
#28269=DIRECTION('',(0.,-0.499999999999997,-0.866025403784441));
#28270=DIRECTION('',(1.,0.,0.));
#28271=DIRECTION('center_axis',(0.,-3.00462919747432E-15,1.));
#28272=DIRECTION('ref_axis',(0.,-1.,-3.00462919747432E-15));
#28273=DIRECTION('',(0.,-1.,-3.00462919747432E-15));
#28274=DIRECTION('',(0.,-1.,-3.00462919747432E-15));
#28275=DIRECTION('',(1.,0.,0.));
#28276=DIRECTION('center_axis',(0.,0.866025403784434,0.500000000000008));
#28277=DIRECTION('ref_axis',(0.,-0.500000000000007,0.866025403784434));
#28278=DIRECTION('',(0.,-0.500000000000008,0.866025403784434));
#28279=DIRECTION('',(0.,-0.500000000000008,0.866025403784434));
#28280=DIRECTION('',(1.,0.,0.));
#28281=DIRECTION('center_axis',(0.,0.86602540378444,-0.499999999999998));
#28282=DIRECTION('ref_axis',(0.,0.499999999999998,0.86602540378444));
#28283=DIRECTION('',(0.,0.499999999999998,0.86602540378444));
#28284=DIRECTION('',(0.,0.499999999999998,0.86602540378444));
#28285=DIRECTION('',(1.,0.,0.));
#28286=DIRECTION('center_axis',(0.,3.00462919747432E-15,-1.));
#28287=DIRECTION('ref_axis',(0.,1.,3.00462919747432E-15));
#28288=DIRECTION('',(0.,1.,3.00462919747432E-15));
#28289=DIRECTION('',(0.,1.,3.00462919747432E-15));
#28290=DIRECTION('center_axis',(1.,0.,0.));
#28291=DIRECTION('ref_axis',(0.,0.,-1.));
#28292=DIRECTION('center_axis',(1.,0.,0.));
#28293=DIRECTION('ref_axis',(0.,0.,-1.));
#28294=DIRECTION('center_axis',(1.,0.,0.));
#28295=DIRECTION('ref_axis',(0.,0.,-1.));
#28296=DIRECTION('center_axis',(1.,0.,0.));
#28297=DIRECTION('ref_axis',(0.,0.,-1.));
#28298=DIRECTION('center_axis',(1.,0.,0.));
#28299=DIRECTION('ref_axis',(0.,0.,-1.));
#28300=DIRECTION('center_axis',(1.,0.,0.));
#28301=DIRECTION('ref_axis',(0.,0.,-1.));
#28302=DIRECTION('center_axis',(0.,-0.866025403784439,-0.499999999999999));
#28303=DIRECTION('ref_axis',(0.,0.499999999999999,-0.866025403784439));
#28304=DIRECTION('',(1.,0.,0.));
#28305=DIRECTION('',(0.,0.499999999999999,-0.866025403784439));
#28306=DIRECTION('',(0.,0.499999999999999,-0.866025403784439));
#28307=DIRECTION('',(1.,0.,0.));
#28308=DIRECTION('center_axis',(0.,-0.866025403784438,0.500000000000002));
#28309=DIRECTION('ref_axis',(0.,-0.500000000000002,-0.866025403784438));
#28310=DIRECTION('',(0.,-0.500000000000002,-0.866025403784438));
#28311=DIRECTION('',(0.,-0.500000000000002,-0.866025403784438));
#28312=DIRECTION('',(1.,0.,0.));
#28313=DIRECTION('center_axis',(0.,1.00154306582478E-15,1.));
#28314=DIRECTION('ref_axis',(0.,-1.,1.00154306582478E-15));
#28315=DIRECTION('',(0.,-1.,1.00154306582478E-15));
#28316=DIRECTION('',(0.,-1.,1.00154306582478E-15));
#28317=DIRECTION('',(1.,0.,0.));
#28318=DIRECTION('center_axis',(0.,0.866025403784439,0.499999999999999));
#28319=DIRECTION('ref_axis',(0.,-0.499999999999999,0.866025403784439));
#28320=DIRECTION('',(0.,-0.499999999999999,0.866025403784439));
#28321=DIRECTION('',(0.,-0.499999999999999,0.866025403784439));
#28322=DIRECTION('',(1.,0.,0.));
#28323=DIRECTION('center_axis',(0.,0.866025403784438,-0.500000000000002));
#28324=DIRECTION('ref_axis',(0.,0.500000000000002,0.866025403784438));
#28325=DIRECTION('',(0.,0.500000000000002,0.866025403784438));
#28326=DIRECTION('',(0.,0.500000000000002,0.866025403784438));
#28327=DIRECTION('',(1.,0.,0.));
#28328=DIRECTION('center_axis',(0.,-1.00154306582478E-15,-1.));
#28329=DIRECTION('ref_axis',(0.,1.,-1.00154306582478E-15));
#28330=DIRECTION('',(0.,1.,-1.00154306582478E-15));
#28331=DIRECTION('',(0.,1.,-1.00154306582478E-15));
#28332=DIRECTION('center_axis',(1.,0.,0.));
#28333=DIRECTION('ref_axis',(0.,0.,-1.));
#28334=DIRECTION('center_axis',(1.,0.,0.));
#28335=DIRECTION('ref_axis',(0.,0.,-1.));
#28336=DIRECTION('center_axis',(1.,0.,0.));
#28337=DIRECTION('ref_axis',(0.,0.,-1.));
#28338=DIRECTION('center_axis',(1.,0.,0.));
#28339=DIRECTION('ref_axis',(0.,0.,-1.));
#28340=DIRECTION('center_axis',(1.,0.,0.));
#28341=DIRECTION('ref_axis',(0.,0.,-1.));
#28342=DIRECTION('center_axis',(1.,0.,0.));
#28343=DIRECTION('ref_axis',(0.,0.,-1.));
#28344=DIRECTION('center_axis',(0.,-0.866025403784439,-0.5));
#28345=DIRECTION('ref_axis',(0.,0.5,-0.866025403784439));
#28346=DIRECTION('',(1.,0.,0.));
#28347=DIRECTION('',(0.,0.5,-0.866025403784439));
#28348=DIRECTION('',(0.,0.5,-0.866025403784439));
#28349=DIRECTION('',(1.,0.,0.));
#28350=DIRECTION('center_axis',(0.,-0.866025403784438,0.500000000000002));
#28351=DIRECTION('ref_axis',(0.,-0.500000000000002,-0.866025403784438));
#28352=DIRECTION('',(0.,-0.500000000000002,-0.866025403784438));
#28353=DIRECTION('',(0.,-0.500000000000002,-0.866025403784438));
#28354=DIRECTION('',(1.,0.,0.));
#28355=DIRECTION('center_axis',(0.,1.00154306582477E-15,1.));
#28356=DIRECTION('ref_axis',(0.,-1.,1.00154306582477E-15));
#28357=DIRECTION('',(0.,-1.,1.00154306582477E-15));
#28358=DIRECTION('',(0.,-1.,1.00154306582477E-15));
#28359=DIRECTION('',(1.,0.,0.));
#28360=DIRECTION('center_axis',(0.,0.866025403784439,0.499999999999999));
#28361=DIRECTION('ref_axis',(0.,-0.499999999999999,0.866025403784439));
#28362=DIRECTION('',(0.,-0.499999999999999,0.866025403784439));
#28363=DIRECTION('',(0.,-0.499999999999999,0.866025403784439));
#28364=DIRECTION('',(1.,0.,0.));
#28365=DIRECTION('center_axis',(0.,0.866025403784438,-0.5));
#28366=DIRECTION('ref_axis',(0.,0.5,0.866025403784438));
#28367=DIRECTION('',(0.,0.5,0.866025403784438));
#28368=DIRECTION('',(0.,0.5,0.866025403784438));
#28369=DIRECTION('',(1.,0.,0.));
#28370=DIRECTION('center_axis',(0.,-1.00154306582477E-15,-1.));
#28371=DIRECTION('ref_axis',(0.,1.,-1.00154306582477E-15));
#28372=DIRECTION('',(0.,1.,-1.00154306582477E-15));
#28373=DIRECTION('',(0.,1.,-1.00154306582477E-15));
#28374=DIRECTION('center_axis',(1.,0.,0.));
#28375=DIRECTION('ref_axis',(0.,0.,-1.));
#28376=DIRECTION('center_axis',(1.,0.,0.));
#28377=DIRECTION('ref_axis',(0.,0.,-1.));
#28378=DIRECTION('center_axis',(1.,0.,0.));
#28379=DIRECTION('ref_axis',(0.,0.,-1.));
#28380=DIRECTION('center_axis',(1.,0.,0.));
#28381=DIRECTION('ref_axis',(0.,0.,-1.));
#28382=DIRECTION('center_axis',(1.,0.,0.));
#28383=DIRECTION('ref_axis',(0.,0.,-1.));
#28384=DIRECTION('center_axis',(1.,0.,0.));
#28385=DIRECTION('ref_axis',(0.,0.,-1.));
#28386=DIRECTION('center_axis',(1.,0.,0.));
#28387=DIRECTION('ref_axis',(0.,0.,-1.));
#28388=DIRECTION('center_axis',(1.,0.,0.));
#28389=DIRECTION('ref_axis',(0.,0.,-1.));
#28390=DIRECTION('center_axis',(-1.,0.,0.));
#28391=DIRECTION('ref_axis',(0.,0.,1.));
#28392=DIRECTION('center_axis',(-1.,0.,0.));
#28393=DIRECTION('ref_axis',(0.,0.,1.));
#35178=CARTESIAN_POINT('',(0.,0.,0.));
#35179=CARTESIAN_POINT('Origin',(12.,24.,26.));
#35180=CARTESIAN_POINT('',(12.,-1.77635683940025E-14,21.5));
#35181=CARTESIAN_POINT('Origin',(12.,-1.73472347597681E-14,26.));
#35182=CARTESIAN_POINT('',(12.,24.,21.5));
#35183=CARTESIAN_POINT('',(12.,24.,21.5));
#35184=CARTESIAN_POINT('Origin',(12.,24.,26.));
#35185=CARTESIAN_POINT('Origin',(12.,24.,-26.));
#35186=CARTESIAN_POINT('',(12.,-4.44089209850063E-15,-30.5));
#35187=CARTESIAN_POINT('Origin',(12.,-3.46944695195361E-15,-26.));
#35188=CARTESIAN_POINT('',(12.,24.,-30.5));
#35189=CARTESIAN_POINT('',(12.,24.,-30.5));
#35190=CARTESIAN_POINT('Origin',(12.,24.,-26.));
#35191=CARTESIAN_POINT('Origin',(30.,25.,0.));
#35192=CARTESIAN_POINT('',(24.,25.,12.));
#35193=CARTESIAN_POINT('Origin',(24.,25.,0.));
#35194=CARTESIAN_POINT('',(30.,25.,12.));
#35195=CARTESIAN_POINT('',(30.,25.,12.));
#35196=CARTESIAN_POINT('Origin',(30.,25.,0.));
#35197=CARTESIAN_POINT('Origin',(30.,25.,0.));
#35198=CARTESIAN_POINT('',(22.,25.,7.75));
#35199=CARTESIAN_POINT('Origin',(22.,25.,0.));
#35200=CARTESIAN_POINT('',(24.,25.,7.75));
#35201=CARTESIAN_POINT('',(30.,25.,7.75));
#35202=CARTESIAN_POINT('Origin',(24.,25.,0.));
#35203=CARTESIAN_POINT('Origin',(30.,25.,0.));
#35204=CARTESIAN_POINT('',(6.,25.,6.00000000000001));
#35205=CARTESIAN_POINT('Origin',(6.,25.,0.));
#35206=CARTESIAN_POINT('',(22.,25.,6.00000000000001));
#35207=CARTESIAN_POINT('',(30.,25.,6.00000000000001));
#35208=CARTESIAN_POINT('Origin',(22.,25.,0.));
#35209=CARTESIAN_POINT('Origin',(30.,25.,0.));
#35210=CARTESIAN_POINT('',(3.,25.,7.74999999999999));
#35211=CARTESIAN_POINT('Origin',(3.,25.,0.));
#35212=CARTESIAN_POINT('',(6.,25.,7.74999999999999));
#35213=CARTESIAN_POINT('',(30.,25.,7.74999999999999));
#35214=CARTESIAN_POINT('Origin',(6.,25.,0.));
#35215=CARTESIAN_POINT('Origin',(30.,25.,0.));
#35216=CARTESIAN_POINT('',(0.,25.,12.));
#35217=CARTESIAN_POINT('Origin',(0.,25.,0.));
#35218=CARTESIAN_POINT('',(3.,25.,12.));
#35219=CARTESIAN_POINT('',(30.,25.,12.));
#35220=CARTESIAN_POINT('Origin',(3.,25.,0.));
#35221=CARTESIAN_POINT('Origin',(27.,11.95,-13.05));
#35222=CARTESIAN_POINT('',(26.0987090714587,11.95,-13.05));
#35223=CARTESIAN_POINT('',(27.,11.95,-11.55));
#35224=CARTESIAN_POINT('',(27.,11.95,-11.55));
#35225=CARTESIAN_POINT('',(27.,10.6509618943234,-12.3));
#35226=CARTESIAN_POINT('Origin',(27.,11.95,-13.05));
#35227=CARTESIAN_POINT('',(27.,10.6509618943234,-13.8));
#35228=CARTESIAN_POINT('Origin',(27.,11.95,-13.05));
#35229=CARTESIAN_POINT('',(27.,11.95,-14.55));
#35230=CARTESIAN_POINT('Origin',(27.,11.95,-13.05));
#35231=CARTESIAN_POINT('',(27.,13.2490381056767,-13.8));
#35232=CARTESIAN_POINT('Origin',(27.,11.95,-13.05));
#35233=CARTESIAN_POINT('',(27.,13.2490381056767,-12.3));
#35234=CARTESIAN_POINT('Origin',(27.,11.95,-13.05));
#35235=CARTESIAN_POINT('Origin',(27.,11.95,-13.05));
#35236=CARTESIAN_POINT('Origin',(27.,11.95,13.05));
#35237=CARTESIAN_POINT('',(26.0987090714587,11.95,13.05));
#35238=CARTESIAN_POINT('',(27.,11.95,14.55));
#35239=CARTESIAN_POINT('',(27.,11.95,14.55));
#35240=CARTESIAN_POINT('',(27.,10.6509618943234,13.8));
#35241=CARTESIAN_POINT('Origin',(27.,11.95,13.05));
#35242=CARTESIAN_POINT('',(27.,10.6509618943234,12.3));
#35243=CARTESIAN_POINT('Origin',(27.,11.95,13.05));
#35244=CARTESIAN_POINT('',(27.,11.95,11.55));
#35245=CARTESIAN_POINT('Origin',(27.,11.95,13.05));
#35246=CARTESIAN_POINT('',(27.,13.2490381056767,12.3));
#35247=CARTESIAN_POINT('Origin',(27.,11.95,13.05));
#35248=CARTESIAN_POINT('',(27.,13.2490381056767,13.8));
#35249=CARTESIAN_POINT('Origin',(27.,11.95,13.05));
#35250=CARTESIAN_POINT('Origin',(27.,11.95,13.05));
#35251=CARTESIAN_POINT('Origin',(27.,38.05,-13.05));
#35252=CARTESIAN_POINT('',(26.0987090714587,38.05,-13.05));
#35253=CARTESIAN_POINT('',(27.,38.05,-11.55));
#35254=CARTESIAN_POINT('',(27.,38.05,-11.55));
#35255=CARTESIAN_POINT('',(27.,36.7509618943233,-12.3));
#35256=CARTESIAN_POINT('Origin',(27.,38.05,-13.05));
#35257=CARTESIAN_POINT('',(27.,36.7509618943233,-13.8));
#35258=CARTESIAN_POINT('Origin',(27.,38.05,-13.05));
#35259=CARTESIAN_POINT('',(27.,38.05,-14.55));
#35260=CARTESIAN_POINT('Origin',(27.,38.05,-13.05));
#35261=CARTESIAN_POINT('',(27.,39.3490381056766,-13.8));
#35262=CARTESIAN_POINT('Origin',(27.,38.05,-13.05));
#35263=CARTESIAN_POINT('',(27.,39.3490381056766,-12.3));
#35264=CARTESIAN_POINT('Origin',(27.,38.05,-13.05));
#35265=CARTESIAN_POINT('Origin',(27.,38.05,-13.05));
#35266=CARTESIAN_POINT('Origin',(27.,38.05,13.05));
#35267=CARTESIAN_POINT('',(26.0987090714587,38.05,13.05));
#35268=CARTESIAN_POINT('',(27.,38.05,14.55));
#35269=CARTESIAN_POINT('',(27.,38.05,14.55));
#35270=CARTESIAN_POINT('',(27.,36.7509618943233,13.8));
#35271=CARTESIAN_POINT('Origin',(27.,38.05,13.05));
#35272=CARTESIAN_POINT('',(27.,36.7509618943233,12.3));
#35273=CARTESIAN_POINT('Origin',(27.,38.05,13.05));
#35274=CARTESIAN_POINT('',(27.,38.05,11.55));
#35275=CARTESIAN_POINT('Origin',(27.,38.05,13.05));
#35276=CARTESIAN_POINT('',(27.,39.3490381056766,12.3));
#35277=CARTESIAN_POINT('Origin',(27.,38.05,13.05));
#35278=CARTESIAN_POINT('',(27.,39.3490381056766,13.8));
#35279=CARTESIAN_POINT('Origin',(27.,38.05,13.05));
#35280=CARTESIAN_POINT('Origin',(27.,38.05,13.05));
#35281=CARTESIAN_POINT('Origin',(30.,11.95,13.05));
#35282=CARTESIAN_POINT('',(24.,11.95,9.94999999999999));
#35283=CARTESIAN_POINT('Origin',(24.,11.95,13.05));
#35284=CARTESIAN_POINT('',(30.,11.95,9.94999999999999));
#35285=CARTESIAN_POINT('',(30.,11.95,9.94999999999999));
#35286=CARTESIAN_POINT('Origin',(30.,11.95,13.05));
#35287=CARTESIAN_POINT('Origin',(30.,11.95,-13.05));
#35288=CARTESIAN_POINT('',(24.,11.95,-16.15));
#35289=CARTESIAN_POINT('Origin',(24.,11.95,-13.05));
#35290=CARTESIAN_POINT('',(30.,11.95,-16.15));
#35291=CARTESIAN_POINT('',(30.,11.95,-16.15));
#35292=CARTESIAN_POINT('Origin',(30.,11.95,-13.05));
#35293=CARTESIAN_POINT('Origin',(30.,38.05,-13.05));
#35294=CARTESIAN_POINT('',(24.,38.05,-16.15));
#35295=CARTESIAN_POINT('Origin',(24.,38.05,-13.05));
#35296=CARTESIAN_POINT('',(30.,38.05,-16.15));
#35297=CARTESIAN_POINT('',(30.,38.05,-16.15));
#35298=CARTESIAN_POINT('Origin',(30.,38.05,-13.05));
#35299=CARTESIAN_POINT('Origin',(30.,38.05,13.05));
#35300=CARTESIAN_POINT('',(24.,38.05,9.94999999999999));
#35301=CARTESIAN_POINT('Origin',(24.,38.05,13.05));
#35302=CARTESIAN_POINT('',(30.,38.05,9.94999999999999));
#35303=CARTESIAN_POINT('',(30.,38.05,9.94999999999999));
#35304=CARTESIAN_POINT('Origin',(30.,38.05,13.05));
#35305=CARTESIAN_POINT('Origin',(30.,11.95,-13.05));
#35306=CARTESIAN_POINT('',(30.,11.95,-16.55));
#35307=CARTESIAN_POINT('Origin',(30.,11.95,-13.05));
#35308=CARTESIAN_POINT('',(24.,11.95,-16.55));
#35309=CARTESIAN_POINT('',(30.,11.95,-16.55));
#35310=CARTESIAN_POINT('Origin',(24.,11.95,-13.05));
#35311=CARTESIAN_POINT('Origin',(30.,11.95,13.05));
#35312=CARTESIAN_POINT('',(30.,11.95,9.55));
#35313=CARTESIAN_POINT('Origin',(30.,11.95,13.05));
#35314=CARTESIAN_POINT('',(24.,11.95,9.55));
#35315=CARTESIAN_POINT('',(30.,11.95,9.55));
#35316=CARTESIAN_POINT('Origin',(24.,11.95,13.05));
#35317=CARTESIAN_POINT('Origin',(30.,38.05,-13.05));
#35318=CARTESIAN_POINT('',(30.,38.05,-16.55));
#35319=CARTESIAN_POINT('Origin',(30.,38.05,-13.05));
#35320=CARTESIAN_POINT('',(24.,38.05,-16.55));
#35321=CARTESIAN_POINT('',(30.,38.05,-16.55));
#35322=CARTESIAN_POINT('Origin',(24.,38.05,-13.05));
#35323=CARTESIAN_POINT('Origin',(30.,38.05,13.05));
#35324=CARTESIAN_POINT('',(30.,38.05,9.54999999999998));
#35325=CARTESIAN_POINT('Origin',(30.,38.05,13.05));
#35326=CARTESIAN_POINT('',(24.,38.05,9.54999999999998));
#35327=CARTESIAN_POINT('',(30.,38.05,9.54999999999998));
#35328=CARTESIAN_POINT('Origin',(24.,38.05,13.05));
#35329=CARTESIAN_POINT('Origin',(24.,0.,0.));
#35330=CARTESIAN_POINT('Origin',(24.,0.,0.));
#35331=CARTESIAN_POINT('Origin',(24.,0.,0.));
#35332=CARTESIAN_POINT('Origin',(24.,0.,0.));
#35333=CARTESIAN_POINT('Origin',(24.,0.,0.));
#35334=CARTESIAN_POINT('',(24.,24.,18.0000000000001));
#35335=CARTESIAN_POINT('',(24.,24.,34.5));
#35336=CARTESIAN_POINT('',(24.,24.,18.0000000000001));
#35337=CARTESIAN_POINT('',(24.,23.5,35.));
#35338=CARTESIAN_POINT('',(24.,24.,34.5));
#35339=CARTESIAN_POINT('',(24.,7.70371977754894E-31,35.));
#35340=CARTESIAN_POINT('',(24.,23.5,35.));
#35341=CARTESIAN_POINT('',(24.,1.78732264387927E-14,-35.));
#35342=CARTESIAN_POINT('',(24.,7.70371977754894E-31,35.));
#35343=CARTESIAN_POINT('',(24.,23.5,-35.));
#35344=CARTESIAN_POINT('',(24.,23.5,-35.));
#35345=CARTESIAN_POINT('',(24.,24.,-34.5));
#35346=CARTESIAN_POINT('',(24.,24.,-34.5));
#35347=CARTESIAN_POINT('',(24.,24.,-17.9999999999999));
#35348=CARTESIAN_POINT('',(24.,24.,-17.9999999999999));
#35349=CARTESIAN_POINT('',(24.,42.5,-17.9999999999999));
#35350=CARTESIAN_POINT('',(24.,42.5,-17.9999999999999));
#35351=CARTESIAN_POINT('',(24.,43.,-17.4999999999999));
#35352=CARTESIAN_POINT('',(24.,43.,-17.4999999999999));
#35353=CARTESIAN_POINT('',(24.,43.,17.5));
#35354=CARTESIAN_POINT('',(24.,43.,17.5));
#35355=CARTESIAN_POINT('',(24.,42.5,18.0000000000001));
#35356=CARTESIAN_POINT('',(24.,42.5,18.0000000000001));
#35357=CARTESIAN_POINT('',(24.,42.5,18.0000000000001));
#35358=CARTESIAN_POINT('',(24.,42.75,15.75));
#35359=CARTESIAN_POINT('',(24.,40.75,17.75));
#35360=CARTESIAN_POINT('',(24.,40.75,17.75));
#35361=CARTESIAN_POINT('',(24.,42.75,-15.75));
#35362=CARTESIAN_POINT('',(24.,42.75,15.75));
#35363=CARTESIAN_POINT('',(24.,40.75,-17.75));
#35364=CARTESIAN_POINT('',(24.,42.75,-15.75));
#35365=CARTESIAN_POINT('',(24.,9.25000000000001,-17.75));
#35366=CARTESIAN_POINT('',(24.,40.75,-17.75));
#35367=CARTESIAN_POINT('',(24.,7.25000000000001,-15.75));
#35368=CARTESIAN_POINT('',(24.,9.25000000000001,-17.75));
#35369=CARTESIAN_POINT('',(24.,7.25000000000001,15.75));
#35370=CARTESIAN_POINT('',(24.,7.25000000000001,15.75));
#35371=CARTESIAN_POINT('',(24.,9.25000000000001,17.75));
#35372=CARTESIAN_POINT('',(24.,9.25000000000001,17.75));
#35373=CARTESIAN_POINT('',(24.,40.75,17.75));
#35374=CARTESIAN_POINT('Origin',(24.,24.,18.0000000000001));
#35375=CARTESIAN_POINT('',(0.,24.,18.0000000000001));
#35376=CARTESIAN_POINT('',(0.,24.,34.5));
#35377=CARTESIAN_POINT('',(0.,24.,18.0000000000001));
#35378=CARTESIAN_POINT('',(24.,24.,34.5));
#35379=CARTESIAN_POINT('',(24.,24.,18.0000000000001));
#35380=CARTESIAN_POINT('Origin',(24.,24.,34.5));
#35381=CARTESIAN_POINT('',(0.,23.5,35.));
#35382=CARTESIAN_POINT('',(0.,24.,34.5));
#35383=CARTESIAN_POINT('',(24.,23.5,35.));
#35384=CARTESIAN_POINT('Origin',(24.,23.5,35.));
#35385=CARTESIAN_POINT('',(0.,7.70371977754894E-31,35.));
#35386=CARTESIAN_POINT('',(0.,23.5,35.));
#35387=CARTESIAN_POINT('',(24.,7.70371977754894E-31,35.));
#35388=CARTESIAN_POINT('Origin',(24.,7.70371977754894E-31,35.));
#35389=CARTESIAN_POINT('',(0.,1.78732264387927E-14,-35.));
#35390=CARTESIAN_POINT('',(0.,7.70371977754894E-31,35.));
#35391=CARTESIAN_POINT('',(24.,1.78732264387927E-14,-35.));
#35392=CARTESIAN_POINT('Origin',(24.,23.5,-35.));
#35393=CARTESIAN_POINT('',(0.,23.5,-35.));
#35394=CARTESIAN_POINT('',(0.,23.5,-35.));
#35395=CARTESIAN_POINT('',(24.,23.5,-35.));
#35396=CARTESIAN_POINT('Origin',(24.,24.,-34.5));
#35397=CARTESIAN_POINT('',(0.,24.,-34.5));
#35398=CARTESIAN_POINT('',(0.,24.,-34.5));
#35399=CARTESIAN_POINT('',(24.,24.,-34.5));
#35400=CARTESIAN_POINT('Origin',(24.,24.,-17.9999999999999));
#35401=CARTESIAN_POINT('',(0.,24.,-17.9999999999999));
#35402=CARTESIAN_POINT('',(0.,24.,-17.9999999999999));
#35403=CARTESIAN_POINT('',(24.,24.,-17.9999999999999));
#35404=CARTESIAN_POINT('Origin',(24.,42.5,-17.9999999999999));
#35405=CARTESIAN_POINT('',(0.,42.5,-17.9999999999999));
#35406=CARTESIAN_POINT('',(0.,42.5,-17.9999999999999));
#35407=CARTESIAN_POINT('',(24.,42.5,-17.9999999999999));
#35408=CARTESIAN_POINT('Origin',(24.,43.,-17.4999999999999));
#35409=CARTESIAN_POINT('',(0.,43.,-17.4999999999999));
#35410=CARTESIAN_POINT('',(0.,43.,-17.4999999999999));
#35411=CARTESIAN_POINT('',(24.,43.,-17.4999999999999));
#35412=CARTESIAN_POINT('Origin',(24.,43.,17.5));
#35413=CARTESIAN_POINT('',(0.,43.,17.5));
#35414=CARTESIAN_POINT('',(0.,43.,17.5));
#35415=CARTESIAN_POINT('',(24.,43.,17.5));
#35416=CARTESIAN_POINT('Origin',(24.,42.5,18.0000000000001));
#35417=CARTESIAN_POINT('',(0.,42.5,18.0000000000001));
#35418=CARTESIAN_POINT('',(0.,42.5,18.0000000000001));
#35419=CARTESIAN_POINT('',(24.,42.5,18.0000000000001));
#35420=CARTESIAN_POINT('Origin',(24.,42.5,18.0000000000001));
#35421=CARTESIAN_POINT('',(0.,42.5,18.0000000000001));
#35422=CARTESIAN_POINT('Origin',(0.,0.,0.));
#35423=CARTESIAN_POINT('Origin',(30.,0.,0.));
#35424=CARTESIAN_POINT('',(30.,42.75,-15.75));
#35425=CARTESIAN_POINT('',(30.,42.75,15.75));
#35426=CARTESIAN_POINT('',(30.,42.75,15.75));
#35427=CARTESIAN_POINT('',(30.,40.75,17.75));
#35428=CARTESIAN_POINT('',(30.,40.75,17.75));
#35429=CARTESIAN_POINT('',(30.,9.25000000000001,17.75));
#35430=CARTESIAN_POINT('',(30.,40.75,17.75));
#35431=CARTESIAN_POINT('',(30.,7.25000000000001,15.75));
#35432=CARTESIAN_POINT('',(30.,9.25000000000001,17.75));
#35433=CARTESIAN_POINT('',(30.,7.25000000000001,-15.75));
#35434=CARTESIAN_POINT('',(30.,7.25000000000001,15.75));
#35435=CARTESIAN_POINT('',(30.,9.25000000000001,-17.75));
#35436=CARTESIAN_POINT('',(30.,9.25000000000001,-17.75));
#35437=CARTESIAN_POINT('',(30.,40.75,-17.75));
#35438=CARTESIAN_POINT('',(30.,40.75,-17.75));
#35439=CARTESIAN_POINT('',(30.,42.75,-15.75));
#35440=CARTESIAN_POINT('Origin',(30.,42.75,15.75));
#35441=CARTESIAN_POINT('',(30.,42.75,15.75));
#35442=CARTESIAN_POINT('',(30.,42.75,-15.75));
#35443=CARTESIAN_POINT('Origin',(30.,40.75,17.75));
#35444=CARTESIAN_POINT('',(30.,40.75,17.75));
#35445=CARTESIAN_POINT('Origin',(30.,40.75,17.75));
#35446=CARTESIAN_POINT('',(30.,9.25000000000001,17.75));
#35447=CARTESIAN_POINT('Origin',(30.,9.25000000000001,17.75));
#35448=CARTESIAN_POINT('',(30.,7.25000000000001,15.75));
#35449=CARTESIAN_POINT('Origin',(30.,7.25000000000001,15.75));
#35450=CARTESIAN_POINT('',(30.,7.25000000000001,-15.75));
#35451=CARTESIAN_POINT('Origin',(30.,9.25000000000001,-17.75));
#35452=CARTESIAN_POINT('',(30.,9.25000000000001,-17.75));
#35453=CARTESIAN_POINT('Origin',(30.,40.75,-17.75));
#35454=CARTESIAN_POINT('',(30.,40.75,-17.75));
#35455=CARTESIAN_POINT('Origin',(30.,42.75,-15.75));
#35456=CARTESIAN_POINT('Origin',(30.,38.05,13.05));
#35457=CARTESIAN_POINT('',(30.,39.7820508075689,13.05));
#35458=CARTESIAN_POINT('',(30.,38.9160254037844,14.55));
#35459=CARTESIAN_POINT('',(30.,39.7820508075689,13.05));
#35460=CARTESIAN_POINT('',(30.,38.9160254037844,11.55));
#35461=CARTESIAN_POINT('',(30.,38.9160254037844,11.55));
#35462=CARTESIAN_POINT('',(30.,37.1839745962155,11.55));
#35463=CARTESIAN_POINT('',(30.,37.1839745962155,11.55));
#35464=CARTESIAN_POINT('',(30.,36.3179491924311,13.05));
#35465=CARTESIAN_POINT('',(30.,36.3179491924311,13.05));
#35466=CARTESIAN_POINT('',(30.,37.1839745962155,14.55));
#35467=CARTESIAN_POINT('',(30.,37.1839745962155,14.55));
#35468=CARTESIAN_POINT('',(30.,38.9160254037844,14.55));
#35469=CARTESIAN_POINT('Origin',(30.,38.05,-13.05));
#35470=CARTESIAN_POINT('',(30.,38.9160254037844,-11.55));
#35471=CARTESIAN_POINT('',(30.,37.1839745962155,-11.55));
#35472=CARTESIAN_POINT('',(30.,38.9160254037844,-11.55));
#35473=CARTESIAN_POINT('',(30.,39.7820508075689,-13.05));
#35474=CARTESIAN_POINT('',(30.,39.7820508075689,-13.05));
#35475=CARTESIAN_POINT('',(30.,38.9160254037844,-14.55));
#35476=CARTESIAN_POINT('',(30.,38.9160254037844,-14.55));
#35477=CARTESIAN_POINT('',(30.,37.1839745962156,-14.55));
#35478=CARTESIAN_POINT('',(30.,37.1839745962156,-14.55));
#35479=CARTESIAN_POINT('',(30.,36.3179491924311,-13.05));
#35480=CARTESIAN_POINT('',(30.,36.3179491924311,-13.05));
#35481=CARTESIAN_POINT('',(30.,37.1839745962155,-11.55));
#35482=CARTESIAN_POINT('Origin',(30.,11.95,-13.05));
#35483=CARTESIAN_POINT('',(30.,12.8160254037845,-11.55));
#35484=CARTESIAN_POINT('',(30.,11.0839745962156,-11.55));
#35485=CARTESIAN_POINT('',(30.,12.8160254037845,-11.55));
#35486=CARTESIAN_POINT('',(30.,13.6820508075689,-13.05));
#35487=CARTESIAN_POINT('',(30.,13.6820508075689,-13.05));
#35488=CARTESIAN_POINT('',(30.,12.8160254037845,-14.55));
#35489=CARTESIAN_POINT('',(30.,12.8160254037845,-14.55));
#35490=CARTESIAN_POINT('',(30.,11.0839745962156,-14.55));
#35491=CARTESIAN_POINT('',(30.,11.0839745962156,-14.55));
#35492=CARTESIAN_POINT('',(30.,10.2179491924311,-13.05));
#35493=CARTESIAN_POINT('',(30.,10.2179491924311,-13.05));
#35494=CARTESIAN_POINT('',(30.,11.0839745962156,-11.55));
#35495=CARTESIAN_POINT('Origin',(30.,11.95,13.05));
#35496=CARTESIAN_POINT('',(30.,12.8160254037845,14.55));
#35497=CARTESIAN_POINT('',(30.,11.0839745962156,14.55));
#35498=CARTESIAN_POINT('',(30.,12.8160254037845,14.55));
#35499=CARTESIAN_POINT('',(30.,13.6820508075689,13.05));
#35500=CARTESIAN_POINT('',(30.,13.6820508075689,13.05));
#35501=CARTESIAN_POINT('',(30.,12.8160254037844,11.55));
#35502=CARTESIAN_POINT('',(30.,12.8160254037844,11.55));
#35503=CARTESIAN_POINT('',(30.,11.0839745962156,11.55));
#35504=CARTESIAN_POINT('',(30.,11.0839745962156,11.55));
#35505=CARTESIAN_POINT('',(30.,10.2179491924311,13.05));
#35506=CARTESIAN_POINT('',(30.,10.2179491924311,13.05));
#35507=CARTESIAN_POINT('',(30.,11.0839745962156,14.55));
#35508=CARTESIAN_POINT('Origin',(27.,37.1839745962155,14.55));
#35509=CARTESIAN_POINT('',(27.,36.3179491924311,13.05));
#35510=CARTESIAN_POINT('',(27.,36.3179491924311,13.05));
#35511=CARTESIAN_POINT('',(27.,37.1839745962155,14.55));
#35512=CARTESIAN_POINT('',(27.,37.1839745962155,14.55));
#35513=CARTESIAN_POINT('',(27.,37.1839745962155,14.55));
#35514=CARTESIAN_POINT('',(27.,37.1839745962155,14.55));
#35515=CARTESIAN_POINT('Origin',(27.,38.9160254037844,14.55));
#35516=CARTESIAN_POINT('',(27.,38.9160254037844,14.55));
#35517=CARTESIAN_POINT('',(27.,38.9160254037844,14.55));
#35518=CARTESIAN_POINT('',(27.,38.9160254037844,14.55));
#35519=CARTESIAN_POINT('',(27.,38.9160254037844,14.55));
#35520=CARTESIAN_POINT('Origin',(27.,39.7820508075689,13.05));
#35521=CARTESIAN_POINT('',(27.,39.7820508075689,13.05));
#35522=CARTESIAN_POINT('',(27.,39.7820508075689,13.05));
#35523=CARTESIAN_POINT('',(27.,39.7820508075689,13.05));
#35524=CARTESIAN_POINT('',(27.,39.7820508075689,13.05));
#35525=CARTESIAN_POINT('Origin',(27.,38.9160254037844,11.55));
#35526=CARTESIAN_POINT('',(27.,38.9160254037844,11.55));
#35527=CARTESIAN_POINT('',(27.,38.9160254037844,11.55));
#35528=CARTESIAN_POINT('',(27.,38.9160254037844,11.55));
#35529=CARTESIAN_POINT('',(27.,38.9160254037844,11.55));
#35530=CARTESIAN_POINT('Origin',(27.,37.1839745962155,11.55));
#35531=CARTESIAN_POINT('',(27.,37.1839745962155,11.55));
#35532=CARTESIAN_POINT('',(27.,37.1839745962155,11.55));
#35533=CARTESIAN_POINT('',(27.,37.1839745962155,11.55));
#35534=CARTESIAN_POINT('',(27.,37.1839745962155,11.55));
#35535=CARTESIAN_POINT('Origin',(27.,36.3179491924311,13.05));
#35536=CARTESIAN_POINT('',(27.,36.3179491924311,13.05));
#35537=CARTESIAN_POINT('',(27.,36.3179491924311,13.05));
#35538=CARTESIAN_POINT('Origin',(27.,0.,0.));
#35539=CARTESIAN_POINT('Origin',(27.,0.,0.));
#35540=CARTESIAN_POINT('Origin',(27.,0.,0.));
#35541=CARTESIAN_POINT('Origin',(27.,0.,0.));
#35542=CARTESIAN_POINT('Origin',(27.,0.,0.));
#35543=CARTESIAN_POINT('Origin',(27.,0.,0.));
#35544=CARTESIAN_POINT('Origin',(27.,36.3179491924311,-13.05));
#35545=CARTESIAN_POINT('',(27.,37.1839745962156,-14.55));
#35546=CARTESIAN_POINT('',(27.,37.1839745962156,-14.55));
#35547=CARTESIAN_POINT('',(27.,36.3179491924311,-13.05));
#35548=CARTESIAN_POINT('',(27.,36.3179491924311,-13.05));
#35549=CARTESIAN_POINT('',(27.,36.3179491924311,-13.05));
#35550=CARTESIAN_POINT('',(27.,36.3179491924311,-13.05));
#35551=CARTESIAN_POINT('Origin',(27.,37.1839745962155,-11.55));
#35552=CARTESIAN_POINT('',(27.,37.1839745962155,-11.55));
#35553=CARTESIAN_POINT('',(27.,37.1839745962155,-11.55));
#35554=CARTESIAN_POINT('',(27.,37.1839745962155,-11.55));
#35555=CARTESIAN_POINT('',(27.,37.1839745962155,-11.55));
#35556=CARTESIAN_POINT('Origin',(27.,38.9160254037844,-11.55));
#35557=CARTESIAN_POINT('',(27.,38.9160254037844,-11.55));
#35558=CARTESIAN_POINT('',(27.,38.9160254037844,-11.55));
#35559=CARTESIAN_POINT('',(27.,38.9160254037844,-11.55));
#35560=CARTESIAN_POINT('',(27.,38.9160254037844,-11.55));
#35561=CARTESIAN_POINT('Origin',(27.,39.7820508075689,-13.05));
#35562=CARTESIAN_POINT('',(27.,39.7820508075689,-13.05));
#35563=CARTESIAN_POINT('',(27.,39.7820508075689,-13.05));
#35564=CARTESIAN_POINT('',(27.,39.7820508075689,-13.05));
#35565=CARTESIAN_POINT('',(27.,39.7820508075689,-13.05));
#35566=CARTESIAN_POINT('Origin',(27.,38.9160254037844,-14.55));
#35567=CARTESIAN_POINT('',(27.,38.9160254037844,-14.55));
#35568=CARTESIAN_POINT('',(27.,38.9160254037844,-14.55));
#35569=CARTESIAN_POINT('',(27.,38.9160254037844,-14.55));
#35570=CARTESIAN_POINT('',(27.,38.9160254037844,-14.55));
#35571=CARTESIAN_POINT('Origin',(27.,37.1839745962156,-14.55));
#35572=CARTESIAN_POINT('',(27.,37.1839745962156,-14.55));
#35573=CARTESIAN_POINT('',(27.,37.1839745962156,-14.55));
#35574=CARTESIAN_POINT('Origin',(27.,0.,0.));
#35575=CARTESIAN_POINT('Origin',(27.,0.,0.));
#35576=CARTESIAN_POINT('Origin',(27.,0.,0.));
#35577=CARTESIAN_POINT('Origin',(27.,0.,0.));
#35578=CARTESIAN_POINT('Origin',(27.,0.,0.));
#35579=CARTESIAN_POINT('Origin',(27.,0.,0.));
#35580=CARTESIAN_POINT('Origin',(27.,10.2179491924311,13.05));
#35581=CARTESIAN_POINT('',(27.,11.0839745962156,11.55));
#35582=CARTESIAN_POINT('',(27.,11.0839745962156,11.55));
#35583=CARTESIAN_POINT('',(27.,10.2179491924311,13.05));
#35584=CARTESIAN_POINT('',(27.,10.2179491924311,13.05));
#35585=CARTESIAN_POINT('',(27.,10.2179491924311,13.05));
#35586=CARTESIAN_POINT('',(27.,10.2179491924311,13.05));
#35587=CARTESIAN_POINT('Origin',(27.,11.0839745962156,14.55));
#35588=CARTESIAN_POINT('',(27.,11.0839745962156,14.55));
#35589=CARTESIAN_POINT('',(27.,11.0839745962156,14.55));
#35590=CARTESIAN_POINT('',(27.,11.0839745962156,14.55));
#35591=CARTESIAN_POINT('',(27.,11.0839745962156,14.55));
#35592=CARTESIAN_POINT('Origin',(27.,12.8160254037845,14.55));
#35593=CARTESIAN_POINT('',(27.,12.8160254037845,14.55));
#35594=CARTESIAN_POINT('',(27.,12.8160254037845,14.55));
#35595=CARTESIAN_POINT('',(27.,12.8160254037845,14.55));
#35596=CARTESIAN_POINT('',(27.,12.8160254037845,14.55));
#35597=CARTESIAN_POINT('Origin',(27.,13.6820508075689,13.05));
#35598=CARTESIAN_POINT('',(27.,13.6820508075689,13.05));
#35599=CARTESIAN_POINT('',(27.,13.6820508075689,13.05));
#35600=CARTESIAN_POINT('',(27.,13.6820508075689,13.05));
#35601=CARTESIAN_POINT('',(27.,13.6820508075689,13.05));
#35602=CARTESIAN_POINT('Origin',(27.,12.8160254037844,11.55));
#35603=CARTESIAN_POINT('',(27.,12.8160254037844,11.55));
#35604=CARTESIAN_POINT('',(27.,12.8160254037844,11.55));
#35605=CARTESIAN_POINT('',(27.,12.8160254037844,11.55));
#35606=CARTESIAN_POINT('',(27.,12.8160254037844,11.55));
#35607=CARTESIAN_POINT('Origin',(27.,11.0839745962156,11.55));
#35608=CARTESIAN_POINT('',(27.,11.0839745962156,11.55));
#35609=CARTESIAN_POINT('',(27.,11.0839745962156,11.55));
#35610=CARTESIAN_POINT('Origin',(27.,0.,0.));
#35611=CARTESIAN_POINT('Origin',(27.,0.,0.));
#35612=CARTESIAN_POINT('Origin',(27.,0.,0.));
#35613=CARTESIAN_POINT('Origin',(27.,0.,0.));
#35614=CARTESIAN_POINT('Origin',(27.,0.,0.));
#35615=CARTESIAN_POINT('Origin',(27.,0.,0.));
#35616=CARTESIAN_POINT('Origin',(27.,10.2179491924311,-13.05));
#35617=CARTESIAN_POINT('',(27.,11.0839745962156,-14.55));
#35618=CARTESIAN_POINT('',(27.,11.0839745962156,-14.55));
#35619=CARTESIAN_POINT('',(27.,10.2179491924311,-13.05));
#35620=CARTESIAN_POINT('',(27.,10.2179491924311,-13.05));
#35621=CARTESIAN_POINT('',(27.,10.2179491924311,-13.05));
#35622=CARTESIAN_POINT('',(27.,10.2179491924311,-13.05));
#35623=CARTESIAN_POINT('Origin',(27.,11.0839745962156,-11.55));
#35624=CARTESIAN_POINT('',(27.,11.0839745962156,-11.55));
#35625=CARTESIAN_POINT('',(27.,11.0839745962156,-11.55));
#35626=CARTESIAN_POINT('',(27.,11.0839745962156,-11.55));
#35627=CARTESIAN_POINT('',(27.,11.0839745962156,-11.55));
#35628=CARTESIAN_POINT('Origin',(27.,12.8160254037845,-11.55));
#35629=CARTESIAN_POINT('',(27.,12.8160254037845,-11.55));
#35630=CARTESIAN_POINT('',(27.,12.8160254037845,-11.55));
#35631=CARTESIAN_POINT('',(27.,12.8160254037845,-11.55));
#35632=CARTESIAN_POINT('',(27.,12.8160254037845,-11.55));
#35633=CARTESIAN_POINT('Origin',(27.,13.6820508075689,-13.05));
#35634=CARTESIAN_POINT('',(27.,13.6820508075689,-13.05));
#35635=CARTESIAN_POINT('',(27.,13.6820508075689,-13.05));
#35636=CARTESIAN_POINT('',(27.,13.6820508075689,-13.05));
#35637=CARTESIAN_POINT('',(27.,13.6820508075689,-13.05));
#35638=CARTESIAN_POINT('Origin',(27.,12.8160254037845,-14.55));
#35639=CARTESIAN_POINT('',(27.,12.8160254037845,-14.55));
#35640=CARTESIAN_POINT('',(27.,12.8160254037845,-14.55));
#35641=CARTESIAN_POINT('',(27.,12.8160254037845,-14.55));
#35642=CARTESIAN_POINT('',(27.,12.8160254037845,-14.55));
#35643=CARTESIAN_POINT('Origin',(27.,11.0839745962156,-14.55));
#35644=CARTESIAN_POINT('',(27.,11.0839745962156,-14.55));
#35645=CARTESIAN_POINT('',(27.,11.0839745962156,-14.55));
#35646=CARTESIAN_POINT('Origin',(27.,0.,0.));
#35647=CARTESIAN_POINT('Origin',(27.,0.,0.));
#35648=CARTESIAN_POINT('Origin',(27.,0.,0.));
#35649=CARTESIAN_POINT('Origin',(27.,0.,0.));
#35650=CARTESIAN_POINT('Origin',(27.,0.,0.));
#35651=CARTESIAN_POINT('Origin',(27.,0.,0.));
#35652=CARTESIAN_POINT('Origin',(3.,37.,0.));
#35653=CARTESIAN_POINT('Origin',(6.,32.75,0.));
#35654=CARTESIAN_POINT('Origin',(22.,31.,0.));
#35655=CARTESIAN_POINT('Origin',(24.,32.75,0.));
#57009=UNCERTAINTY_MEASURE_WITH_UNIT(LENGTH_MEASURE(0.01),#57080,
'DISTANCE_ACCURACY_VALUE',
'Maximum model space distance between geometric entities at asserted c
onnectivities');
#57040=UNCERTAINTY_MEASURE_WITH_UNIT(LENGTH_MEASURE(0.01),#57080,
'DISTANCE_ACCURACY_VALUE',
'Maximum model space distance between geometric entities at asserted c
onnectivities');
#57048=(
GEOMETRIC_REPRESENTATION_CONTEXT(3)
GLOBAL_UNCERTAINTY_ASSIGNED_CONTEXT((#57009))
GLOBAL_UNIT_ASSIGNED_CONTEXT((#57080,#57082,#57083))
REPRESENTATION_CONTEXT('','3D')
);
#57079=(
GEOMETRIC_REPRESENTATION_CONTEXT(3)
GLOBAL_UNCERTAINTY_ASSIGNED_CONTEXT((#57040))
GLOBAL_UNIT_ASSIGNED_CONTEXT((#57080,#57082,#57083))
REPRESENTATION_CONTEXT('','3D')
);
#57080=(
LENGTH_UNIT()
NAMED_UNIT(*)
SI_UNIT(.MILLI.,.METRE.)
);
#57082=(
NAMED_UNIT(*)
PLANE_ANGLE_UNIT()
SI_UNIT($,.RADIAN.)
);
#57083=(
NAMED_UNIT(*)
SI_UNIT($,.STERADIAN.)
SOLID_ANGLE_UNIT()
);
#57091=SHAPE_DEFINITION_REPRESENTATION(#57131,#57256);
#57131=PRODUCT_DEFINITION_SHAPE('',$,#57295);
#57256=SHAPE_REPRESENTATION('',(#25057),#57048);
#57287=PRODUCT_DEFINITION_CONTEXT('part definition',#57403,'design');
#57295=PRODUCT_DEFINITION('Floating Bearing Housing',
'Floating Bearing Housing',#57333,#57287);
#57333=PRODUCT_DEFINITION_FORMATION('',$,#57412);
#57403=APPLICATION_CONTEXT(
'Core Data for Automotive Mechanical Design Process');
#57404=PRODUCT_CONTEXT('part definition',#57403,'mechanical');
#57412=PRODUCT('Floating Bearing Housing','Floating Bearing Housing',$,
(#57404));
#57444=PRESENTATION_STYLE_ASSIGNMENT((#57446));
#57446=SURFACE_STYLE_USAGE(.BOTH.,#57448);
#57448=SURFACE_SIDE_STYLE('',(#57450));
#57450=SURFACE_STYLE_FILL_AREA(#57452);
#57452=FILL_AREA_STYLE('Opaque(202,209,238)',(#57454));
#57454=FILL_AREA_STYLE_COLOUR('Opaque(202,209,238)',#57456);
#57456=COLOUR_RGB('Opaque(202,209,238)',0.792156862745098,0.819607843137255,
0.933333333333333);
ENDSEC;
END-ISO-10303-21;
